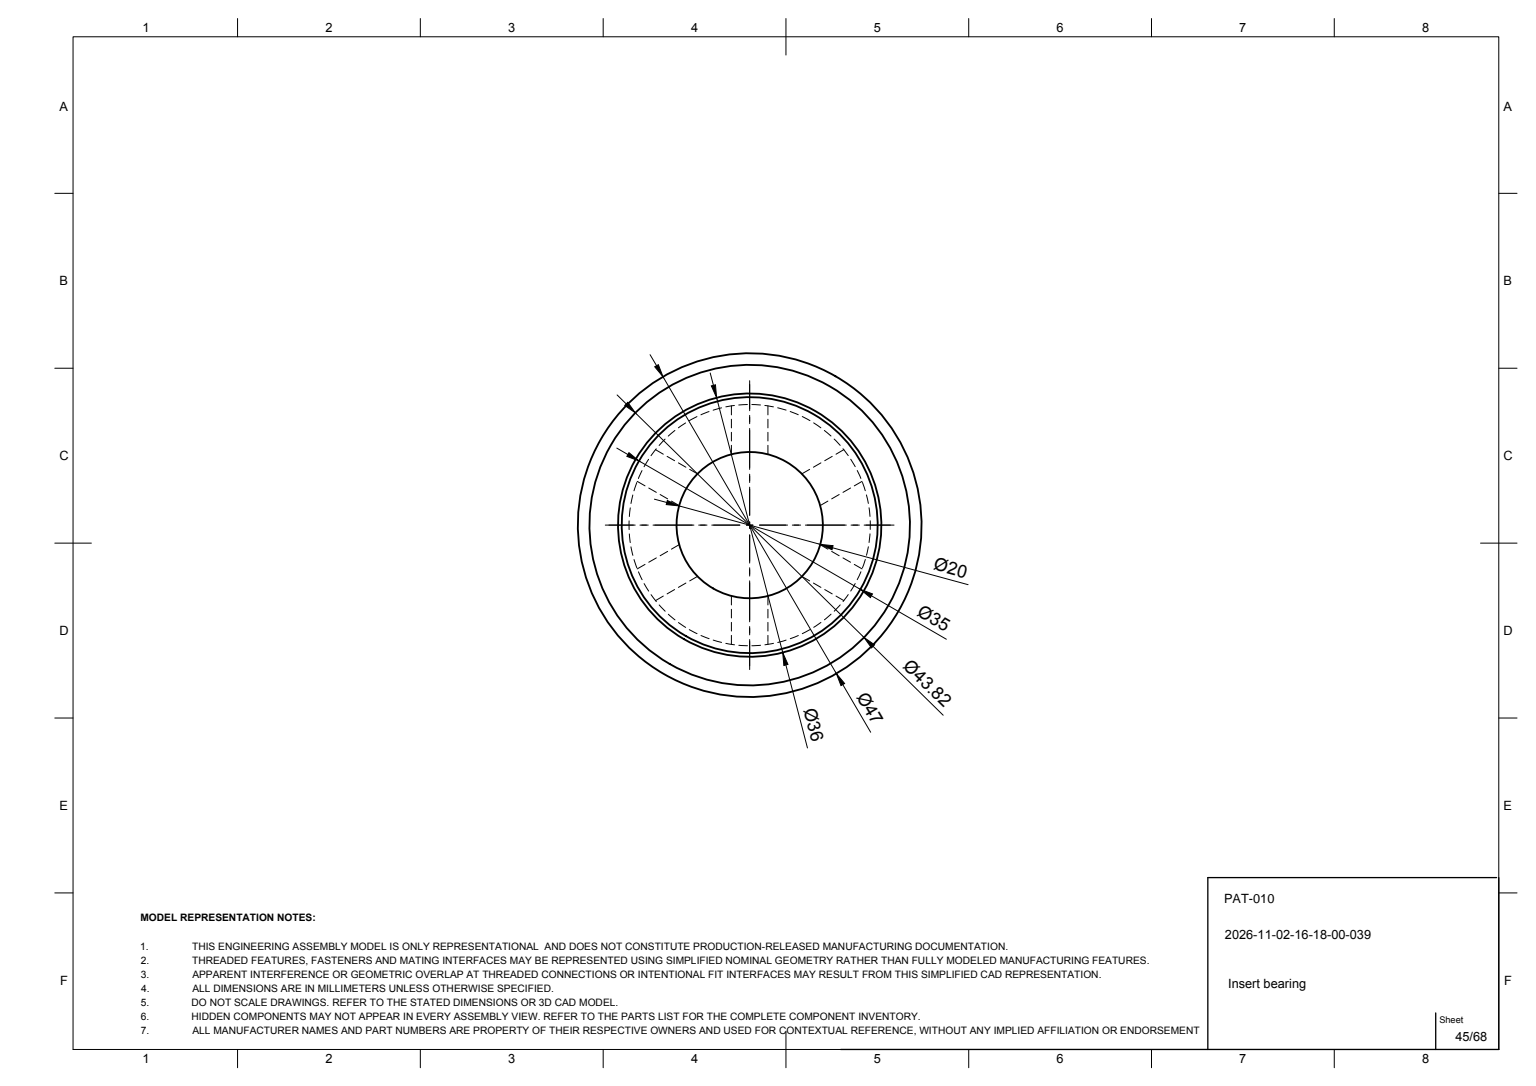
ISO-10303-21;
HEADER;
/* Generated by software containing ST-Developer
 * from STEP Tools, Inc. (www.steptools.com) 
 */

FILE_DESCRIPTION(
/* description */ ('Belt conveyor head drive unit'),
/* implementation_level */ '2;1');

FILE_NAME(
/* name */ 'Insert bearing.step',
/* time_stamp */ '2026-10-28T03:26:19-07:00',
/* author */ (''),
/* organization */ (''),
/* preprocessor_version */ 'ST-DEVELOPER v20.2',
/* originating_system */ 'Autodesk Translation Framework v15.17.0.0',
/* authorisation */ '');

FILE_SCHEMA (('AUTOMOTIVE_DESIGN { 1 0 10303 214 3 1 1 }'));
ENDSEC;

DATA;
#10=MECHANICAL_DESIGN_GEOMETRIC_PRESENTATION_REPRESENTATION('',(#902,#903),#27069);
#553=B_SPLINE_CURVE_WITH_KNOTS('',3,(#23805,#23806,#23807,#23808,#23809,
#23810,#23811,#23812,#23813,#23814),.UNSPECIFIED.,.F.,.F.,(4,2,2,2,4),(1.13193471301885,
1.22626174930539,1.32058878559194,1.41491753480854,1.50924628402513),
 .UNSPECIFIED.);
#554=B_SPLINE_CURVE_WITH_KNOTS('',3,(#23816,#23817,#23818,#23819,#23820,
#23821,#23822,#23823,#23824,#23825,#23826,#23827,#23828,#23829,#23830,#23831,
#23832,#23833),.UNSPECIFIED.,.F.,.F.,(4,2,2,2,2,2,2,2,4),(0.377311571006283,
0.471638607292829,0.565965643579376,0.66029439279597,0.754623142012565,
0.84895189122916,0.943280640445754,1.0376076767323,1.13193471301885),
 .UNSPECIFIED.);
#555=B_SPLINE_CURVE_WITH_KNOTS('',3,(#23834,#23835,#23836,#23837,#23838,
#23839,#23840,#23841,#23842,#23843),.UNSPECIFIED.,.F.,.F.,(4,2,2,2,4),(1.50924628402513,
1.60357503324173,1.69790378245832,1.79223081874487,1.88655785503141),
 .UNSPECIFIED.);
#556=B_SPLINE_CURVE_WITH_KNOTS('',3,(#23846,#23847,#23848,#23849,#23850,
#23851,#23852,#23853,#23854,#23855,#23856,#23857,#23858,#23859,#23860,#23861,
#23862,#23863,#23864,#23865,#23866,#23867,#23868,#23869,#23870,#23871,#23872,
#23873,#23874,#23875,#23876,#23877,#23878,#23879),.UNSPECIFIED.,.T.,.F.,
(4,2,2,2,2,2,2,2,2,2,2,2,2,2,2,2,4),(0.,0.0946120580087934,0.189224116017587,
0.283822945575014,0.378421775132442,0.47302060468987,0.567619434247297,
0.662231492256091,0.756843550264884,0.851455608273677,0.94606766628247,
1.0406664958399,1.13526532539733,1.22986415495475,1.32446298451218,1.41907504252097,
1.51368710052977),.UNSPECIFIED.);
#557=B_SPLINE_CURVE_WITH_KNOTS('',3,(#23882,#23883,#23884,#23885,#23886,
#23887,#23888,#23889,#23890,#23891,#23892,#23893,#23894,#23895,#23896,#23897,
#23898,#23899,#23900,#23901,#23902,#23903,#23904,#23905,#23906,#23907,#23908,
#23909,#23910,#23911,#23912,#23913,#23914,#23915),.UNSPECIFIED.,.T.,.F.,
(4,2,2,2,2,2,2,2,2,2,2,2,2,2,2,2,4),(0.,0.0946120580087934,0.189224116017587,
0.283822945575014,0.378421775132442,0.47302060468987,0.567619434247297,
0.66223149225609,0.756843550264884,0.851455608273677,0.94606766628247,1.0406664958399,
1.13526532539733,1.22986415495475,1.32446298451218,1.41907504252097,1.51368710052977),
 .UNSPECIFIED.);
#558=B_SPLINE_CURVE_WITH_KNOTS('',3,(#23919,#23920,#23921,#23922,#23923,
#23924,#23925,#23926,#23927,#23928),.UNSPECIFIED.,.F.,.F.,(4,2,2,2,4),(1.13193471301885,
1.22626174930539,1.32058878559194,1.41491753480854,1.50924628402513),
 .UNSPECIFIED.);
#559=B_SPLINE_CURVE_WITH_KNOTS('',3,(#23930,#23931,#23932,#23933,#23934,
#23935,#23936,#23937,#23938,#23939,#23940,#23941,#23942,#23943,#23944,#23945,
#23946,#23947),.UNSPECIFIED.,.F.,.F.,(4,2,2,2,2,2,2,2,4),(0.377311571006283,
0.47163860729283,0.565965643579376,0.660294392795971,0.754623142012565,
0.84895189122916,0.943280640445755,1.0376076767323,1.13193471301885),
 .UNSPECIFIED.);
#560=B_SPLINE_CURVE_WITH_KNOTS('',3,(#23948,#23949,#23950,#23951,#23952,
#23953,#23954,#23955,#23956,#23957),.UNSPECIFIED.,.F.,.F.,(4,2,2,2,4),(1.50924628402513,
1.60357503324173,1.69790378245832,1.79223081874487,1.88655785503141),
 .UNSPECIFIED.);
#561=B_SPLINE_CURVE_WITH_KNOTS('',3,(#23966,#23967,#23968,#23969,#23970,
#23971,#23972,#23973,#23974,#23975,#23976,#23977,#23978,#23979,#23980,#23981,
#23982,#23983),.UNSPECIFIED.,.F.,.F.,(4,2,2,2,2,2,2,2,4),(0.377311571006282,
0.471638607292829,0.565965643579376,0.660294392795971,0.754623142012565,
0.84895189122916,0.943280640445754,1.0376076767323,1.13193471301885),
 .UNSPECIFIED.);
#562=B_SPLINE_CURVE_WITH_KNOTS('',3,(#23985,#23986,#23987,#23988,#23989,
#23990,#23991,#23992,#23993,#23994),.UNSPECIFIED.,.F.,.F.,(4,2,2,2,4),(1.13193471301885,
1.22626174930539,1.32058878559194,1.41491753480854,1.50924628402513),
 .UNSPECIFIED.);
#563=B_SPLINE_CURVE_WITH_KNOTS('',3,(#23995,#23996,#23997,#23998,#23999,
#24000,#24001,#24002,#24003,#24004),.UNSPECIFIED.,.F.,.F.,(4,2,2,2,4),(1.50924628402513,
1.60357503324172,1.69790378245832,1.79223081874487,1.88655785503141),
 .UNSPECIFIED.);
#564=B_SPLINE_CURVE_WITH_KNOTS('',3,(#24007,#24008,#24009,#24010,#24011,
#24012,#24013,#24014,#24015,#24016,#24017,#24018,#24019,#24020,#24021,#24022,
#24023,#24024),.UNSPECIFIED.,.F.,.F.,(4,2,2,2,2,2,2,2,4),(0.377311571006283,
0.47163860729283,0.565965643579376,0.660294392795971,0.754623142012565,
0.84895189122916,0.943280640445754,1.0376076767323,1.13193471301885),
 .UNSPECIFIED.);
#565=B_SPLINE_CURVE_WITH_KNOTS('',3,(#24026,#24027,#24028,#24029,#24030,
#24031,#24032,#24033,#24034,#24035),.UNSPECIFIED.,.F.,.F.,(4,2,2,2,4),(1.13193471301885,
1.22626174930539,1.32058878559194,1.41491753480854,1.50924628402513),
 .UNSPECIFIED.);
#566=B_SPLINE_CURVE_WITH_KNOTS('',3,(#24036,#24037,#24038,#24039,#24040,
#24041,#24042,#24043,#24044,#24045),.UNSPECIFIED.,.F.,.F.,(4,2,2,2,4),(1.50924628402513,
1.60357503324173,1.69790378245832,1.79223081874487,1.88655785503141),
 .UNSPECIFIED.);
#567=B_SPLINE_CURVE_WITH_KNOTS('',3,(#24048,#24049,#24050,#24051,#24052,
#24053,#24054,#24055,#24056,#24057,#24058,#24059,#24060,#24061,#24062,#24063,
#24064,#24065),.UNSPECIFIED.,.F.,.F.,(4,2,2,2,2,2,2,2,4),(0.377311571006282,
0.471638607292829,0.565965643579376,0.66029439279597,0.754623142012565,
0.84895189122916,0.943280640445754,1.0376076767323,1.13193471301885),
 .UNSPECIFIED.);
#568=B_SPLINE_CURVE_WITH_KNOTS('',3,(#24067,#24068,#24069,#24070,#24071,
#24072,#24073,#24074,#24075,#24076),.UNSPECIFIED.,.F.,.F.,(4,2,2,2,4),(1.13193471301885,
1.22626174930539,1.32058878559194,1.41491753480854,1.50924628402513),
 .UNSPECIFIED.);
#569=B_SPLINE_CURVE_WITH_KNOTS('',3,(#24077,#24078,#24079,#24080,#24081,
#24082,#24083,#24084,#24085,#24086),.UNSPECIFIED.,.F.,.F.,(4,2,2,2,4),(1.50924628402513,
1.60357503324172,1.69790378245832,1.79223081874487,1.88655785503141),
 .UNSPECIFIED.);
#570=B_SPLINE_CURVE_WITH_KNOTS('',3,(#24089,#24090,#24091,#24092,#24093,
#24094,#24095,#24096,#24097,#24098,#24099,#24100,#24101,#24102,#24103,#24104,
#24105,#24106),.UNSPECIFIED.,.F.,.F.,(4,2,2,2,2,2,2,2,4),(0.377311571006283,
0.471638607292829,0.565965643579376,0.660294392795971,0.754623142012565,
0.84895189122916,0.943280640445755,1.0376076767323,1.13193471301885),
 .UNSPECIFIED.);
#571=B_SPLINE_CURVE_WITH_KNOTS('',3,(#24108,#24109,#24110,#24111,#24112,
#24113,#24114,#24115,#24116,#24117),.UNSPECIFIED.,.F.,.F.,(4,2,2,2,4),(1.13193471301885,
1.22626174930539,1.32058878559194,1.41491753480854,1.50924628402513),
 .UNSPECIFIED.);
#572=B_SPLINE_CURVE_WITH_KNOTS('',3,(#24118,#24119,#24120,#24121,#24122,
#24123,#24124,#24125,#24126,#24127),.UNSPECIFIED.,.F.,.F.,(4,2,2,2,4),(1.50924628402513,
1.60357503324172,1.69790378245832,1.79223081874487,1.88655785503141),
 .UNSPECIFIED.);
#573=B_SPLINE_CURVE_WITH_KNOTS('',3,(#24131,#24132,#24133,#24134,#24135,
#24136,#24137,#24138,#24139,#24140,#24141,#24142,#24143,#24144,#24145,#24146,
#24147,#24148,#24149,#24150,#24151,#24152,#24153,#24154,#24155,#24156,#24157,
#24158,#24159,#24160,#24161,#24162,#24163,#24164),.UNSPECIFIED.,.T.,.F.,
(4,2,2,2,2,2,2,2,2,2,2,2,2,2,2,2,4),(0.,0.0946120580087934,0.189224116017587,
0.283822945575014,0.378421775132442,0.47302060468987,0.567619434247297,
0.66223149225609,0.756843550264884,0.851455608273677,0.94606766628247,1.0406664958399,
1.13526532539733,1.22986415495475,1.32446298451218,1.41907504252097,1.51368710052977),
 .UNSPECIFIED.);
#574=B_SPLINE_CURVE_WITH_KNOTS('',3,(#24167,#24168,#24169,#24170,#24171,
#24172,#24173,#24174,#24175,#24176,#24177,#24178,#24179,#24180,#24181,#24182,
#24183,#24184,#24185,#24186,#24187,#24188,#24189,#24190,#24191,#24192,#24193,
#24194,#24195,#24196,#24197,#24198,#24199,#24200),.UNSPECIFIED.,.T.,.F.,
(4,2,2,2,2,2,2,2,2,2,2,2,2,2,2,2,4),(0.,0.0946120580087934,0.189224116017587,
0.283822945575014,0.378421775132442,0.47302060468987,0.567619434247297,
0.66223149225609,0.756843550264884,0.851455608273677,0.94606766628247,1.0406664958399,
1.13526532539733,1.22986415495475,1.32446298451218,1.41907504252097,1.51368710052977),
 .UNSPECIFIED.);
#575=B_SPLINE_CURVE_WITH_KNOTS('',3,(#24205,#24206,#24207,#24208,#24209,
#24210,#24211,#24212,#24213,#24214,#24215,#24216,#24217,#24218,#24219,#24220,
#24221,#24222,#24223,#24224,#24225,#24226,#24227,#24228,#24229,#24230,#24231,
#24232,#24233,#24234,#24235,#24236,#24237,#24238),.UNSPECIFIED.,.T.,.F.,
(4,2,2,2,2,2,2,2,2,2,2,2,2,2,2,2,4),(0.,0.0946120580087934,0.189224116017587,
0.283822945575014,0.378421775132442,0.47302060468987,0.567619434247297,
0.66223149225609,0.756843550264884,0.851455608273677,0.94606766628247,1.0406664958399,
1.13526532539733,1.22986415495475,1.32446298451218,1.41907504252097,1.51368710052977),
 .UNSPECIFIED.);
#576=B_SPLINE_CURVE_WITH_KNOTS('',3,(#24241,#24242,#24243,#24244,#24245,
#24246,#24247,#24248,#24249,#24250,#24251,#24252,#24253,#24254,#24255,#24256,
#24257,#24258,#24259,#24260,#24261,#24262,#24263,#24264,#24265,#24266,#24267,
#24268,#24269,#24270,#24271,#24272,#24273,#24274),.UNSPECIFIED.,.T.,.F.,
(4,2,2,2,2,2,2,2,2,2,2,2,2,2,2,2,4),(0.,0.0946120580087934,0.189224116017587,
0.283822945575014,0.378421775132442,0.47302060468987,0.567619434247297,
0.66223149225609,0.756843550264884,0.851455608273677,0.94606766628247,1.0406664958399,
1.13526532539733,1.22986415495475,1.32446298451218,1.41907504252097,1.51368710052977),
 .UNSPECIFIED.);
#676=SPHERICAL_SURFACE('',#15555,2.35);
#749=SHAPE_REPRESENTATION_RELATIONSHIP('SRR','None',#27396,#818);
#818=ADVANCED_BREP_SHAPE_REPRESENTATION('',(#985,#986),#27038);
#902=STYLED_ITEM('',(#27797),#985);
#903=STYLED_ITEM('',(#27797),#986);
#985=MANIFOLD_SOLID_BREP('Body1',#13769);
#986=MANIFOLD_SOLID_BREP('Body2',#13770);
#1182=FACE_BOUND('',#3067,.T.);
#1183=FACE_BOUND('',#3069,.T.);
#1184=FACE_BOUND('',#3070,.T.);
#1185=FACE_BOUND('',#3072,.T.);
#1186=FACE_BOUND('',#3076,.T.);
#1187=FACE_BOUND('',#3077,.T.);
#1188=FACE_BOUND('',#3078,.T.);
#1189=FACE_BOUND('',#3079,.T.);
#1190=FACE_BOUND('',#3080,.T.);
#1191=FACE_BOUND('',#3081,.T.);
#1192=FACE_BOUND('',#3087,.T.);
#1193=FACE_BOUND('',#3089,.T.);
#1194=FACE_BOUND('',#3092,.T.);
#1195=FACE_BOUND('',#3094,.T.);
#1196=FACE_BOUND('',#3095,.T.);
#1197=FACE_BOUND('',#3096,.T.);
#1198=FACE_BOUND('',#3097,.T.);
#1199=FACE_BOUND('',#3098,.T.);
#1200=FACE_BOUND('',#3099,.T.);
#1512=PLANE('',#15553);
#1513=PLANE('',#15558);
#1514=PLANE('',#15568);
#1515=PLANE('',#15570);
#1516=PLANE('',#15574);
#2095=FACE_OUTER_BOUND('',#3065,.T.);
#2096=FACE_OUTER_BOUND('',#3066,.T.);
#2097=FACE_OUTER_BOUND('',#3068,.T.);
#2098=FACE_OUTER_BOUND('',#3071,.T.);
#2099=FACE_OUTER_BOUND('',#3073,.T.);
#2100=FACE_OUTER_BOUND('',#3074,.T.);
#2101=FACE_OUTER_BOUND('',#3075,.T.);
#2102=FACE_OUTER_BOUND('',#3082,.T.);
#2103=FACE_OUTER_BOUND('',#3083,.T.);
#2104=FACE_OUTER_BOUND('',#3084,.T.);
#2105=FACE_OUTER_BOUND('',#3085,.T.);
#2106=FACE_OUTER_BOUND('',#3086,.T.);
#2107=FACE_OUTER_BOUND('',#3088,.T.);
#2108=FACE_OUTER_BOUND('',#3090,.T.);
#2109=FACE_OUTER_BOUND('',#3091,.T.);
#2110=FACE_OUTER_BOUND('',#3093,.T.);
#3065=EDGE_LOOP('',(#10938,#10939,#10940,#10941));
#3066=EDGE_LOOP('',(#10942));
#3067=EDGE_LOOP('',(#10943));
#3068=EDGE_LOOP('',(#10944,#10945));
#3069=EDGE_LOOP('',(#10946));
#3070=EDGE_LOOP('',(#10947));
#3071=EDGE_LOOP('',(#10948));
#3072=EDGE_LOOP('',(#10949));
#3073=EDGE_LOOP('',(#10950,#10951,#10952,#10953,#10954,#10955));
#3074=EDGE_LOOP('',(#10956,#10957,#10958,#10959,#10960,#10961));
#3075=EDGE_LOOP('',(#10962,#10963,#10964,#10965));
#3076=EDGE_LOOP('',(#10966,#10967,#10968));
#3077=EDGE_LOOP('',(#10969,#10970,#10971));
#3078=EDGE_LOOP('',(#10972,#10973,#10974));
#3079=EDGE_LOOP('',(#10975,#10976,#10977));
#3080=EDGE_LOOP('',(#10978,#10979,#10980));
#3081=EDGE_LOOP('',(#10981,#10982,#10983));
#3082=EDGE_LOOP('',(#10984,#10985,#10986,#10987,#10988,#10989));
#3083=EDGE_LOOP('',(#10990,#10991,#10992,#10993,#10994,#10995));
#3084=EDGE_LOOP('',(#10996,#10997,#10998,#10999,#11000,#11001));
#3085=EDGE_LOOP('',(#11002,#11003,#11004,#11005,#11006,#11007));
#3086=EDGE_LOOP('',(#11008));
#3087=EDGE_LOOP('',(#11009));
#3088=EDGE_LOOP('',(#11010));
#3089=EDGE_LOOP('',(#11011));
#3090=EDGE_LOOP('',(#11012,#11013,#11014,#11015));
#3091=EDGE_LOOP('',(#11016));
#3092=EDGE_LOOP('',(#11017));
#3093=EDGE_LOOP('',(#11018,#11019,#11020,#11021));
#3094=EDGE_LOOP('',(#11022));
#3095=EDGE_LOOP('',(#11023));
#3096=EDGE_LOOP('',(#11024));
#3097=EDGE_LOOP('',(#11025));
#3098=EDGE_LOOP('',(#11026));
#3099=EDGE_LOOP('',(#11027));
#3986=LINE('',#23790,#4778);
#3987=LINE('',#23845,#4779);
#3988=LINE('',#23917,#4780);
#3989=LINE('',#23962,#4781);
#3990=LINE('',#24130,#4782);
#3991=LINE('',#24201,#4783);
#3992=LINE('',#24204,#4784);
#3993=LINE('',#24275,#4785);
#3994=LINE('',#24285,#4786);
#3995=LINE('',#24290,#4787);
#4778=VECTOR('',#18902,1.8);
#4779=VECTOR('',#18919,0.25);
#4780=VECTOR('',#18922,0.25);
#4781=VECTOR('',#18927,1.65);
#4782=VECTOR('',#18932,0.25);
#4783=VECTOR('',#18935,0.25);
#4784=VECTOR('',#18938,0.25);
#4785=VECTOR('',#18941,0.25);
#4786=VECTOR('',#18954,1.75);
#4787=VECTOR('',#18961,1.);
#5552=CIRCLE('',#15551,1.8);
#5553=CIRCLE('',#15552,1.8);
#5554=CIRCLE('',#15554,2.19089023002066);
#5555=CIRCLE('',#15556,2.35);
#5556=CIRCLE('',#15557,2.19089023002066);
#5557=CIRCLE('',#15562,1.65);
#5558=CIRCLE('',#15563,1.65);
#5559=CIRCLE('',#15569,1.);
#5560=CIRCLE('',#15571,1.75);
#5561=CIRCLE('',#15573,1.75);
#5562=CIRCLE('',#15575,1.);
#6629=VERTEX_POINT('',#23787);
#6630=VERTEX_POINT('',#23789);
#6631=VERTEX_POINT('',#23793);
#6632=VERTEX_POINT('',#23796);
#6633=VERTEX_POINT('',#23797);
#6634=VERTEX_POINT('',#23799);
#6635=VERTEX_POINT('',#23803);
#6636=VERTEX_POINT('',#23804);
#6637=VERTEX_POINT('',#23815);
#6638=VERTEX_POINT('',#23844);
#6639=VERTEX_POINT('',#23881);
#6640=VERTEX_POINT('',#23916);
#6641=VERTEX_POINT('',#23918);
#6642=VERTEX_POINT('',#23929);
#6643=VERTEX_POINT('',#23959);
#6644=VERTEX_POINT('',#23961);
#6645=VERTEX_POINT('',#23964);
#6646=VERTEX_POINT('',#23965);
#6647=VERTEX_POINT('',#23984);
#6648=VERTEX_POINT('',#24005);
#6649=VERTEX_POINT('',#24006);
#6650=VERTEX_POINT('',#24025);
#6651=VERTEX_POINT('',#24046);
#6652=VERTEX_POINT('',#24047);
#6653=VERTEX_POINT('',#24066);
#6654=VERTEX_POINT('',#24087);
#6655=VERTEX_POINT('',#24088);
#6656=VERTEX_POINT('',#24107);
#6657=VERTEX_POINT('',#24129);
#6658=VERTEX_POINT('',#24166);
#6659=VERTEX_POINT('',#24203);
#6660=VERTEX_POINT('',#24240);
#6661=VERTEX_POINT('',#24277);
#6662=VERTEX_POINT('',#24280);
#6663=VERTEX_POINT('',#24283);
#6664=VERTEX_POINT('',#24287);
#8161=EDGE_CURVE('',#6629,#6629,#5552,.T.);
#8162=EDGE_CURVE('',#6629,#6630,#3986,.T.);
#8163=EDGE_CURVE('',#6630,#6630,#5553,.T.);
#8164=EDGE_CURVE('',#6631,#6631,#5554,.T.);
#8165=EDGE_CURVE('',#6632,#6633,#5555,.T.);
#8166=EDGE_CURVE('',#6634,#6634,#5556,.T.);
#8167=EDGE_CURVE('',#6635,#6636,#553,.T.);
#8168=EDGE_CURVE('',#6637,#6635,#554,.T.);
#8169=EDGE_CURVE('',#6636,#6637,#555,.T.);
#8170=EDGE_CURVE('',#6636,#6638,#3987,.T.);
#8171=EDGE_CURVE('',#6638,#6638,#556,.T.);
#8172=EDGE_CURVE('',#6639,#6639,#557,.T.);
#8173=EDGE_CURVE('',#6639,#6640,#3988,.T.);
#8174=EDGE_CURVE('',#6641,#6640,#558,.T.);
#8175=EDGE_CURVE('',#6642,#6641,#559,.T.);
#8176=EDGE_CURVE('',#6640,#6642,#560,.T.);
#8177=EDGE_CURVE('',#6643,#6643,#5557,.T.);
#8178=EDGE_CURVE('',#6643,#6644,#3989,.T.);
#8179=EDGE_CURVE('',#6644,#6644,#5558,.T.);
#8180=EDGE_CURVE('',#6645,#6646,#561,.T.);
#8181=EDGE_CURVE('',#6646,#6647,#562,.T.);
#8182=EDGE_CURVE('',#6647,#6645,#563,.T.);
#8183=EDGE_CURVE('',#6648,#6649,#564,.T.);
#8184=EDGE_CURVE('',#6649,#6650,#565,.T.);
#8185=EDGE_CURVE('',#6650,#6648,#566,.T.);
#8186=EDGE_CURVE('',#6651,#6652,#567,.T.);
#8187=EDGE_CURVE('',#6652,#6653,#568,.T.);
#8188=EDGE_CURVE('',#6653,#6651,#569,.T.);
#8189=EDGE_CURVE('',#6654,#6655,#570,.T.);
#8190=EDGE_CURVE('',#6655,#6656,#571,.T.);
#8191=EDGE_CURVE('',#6656,#6654,#572,.T.);
#8192=EDGE_CURVE('',#6647,#6657,#3990,.T.);
#8193=EDGE_CURVE('',#6657,#6657,#573,.T.);
#8194=EDGE_CURVE('',#6658,#6658,#574,.T.);
#8195=EDGE_CURVE('',#6658,#6650,#3991,.T.);
#8196=EDGE_CURVE('',#6653,#6659,#3992,.T.);
#8197=EDGE_CURVE('',#6659,#6659,#575,.T.);
#8198=EDGE_CURVE('',#6660,#6660,#576,.T.);
#8199=EDGE_CURVE('',#6660,#6656,#3993,.T.);
#8200=EDGE_CURVE('',#6661,#6661,#5559,.T.);
#8201=EDGE_CURVE('',#6662,#6662,#5560,.T.);
#8202=EDGE_CURVE('',#6663,#6663,#5561,.T.);
#8203=EDGE_CURVE('',#6663,#6662,#3994,.T.);
#8204=EDGE_CURVE('',#6664,#6664,#5562,.T.);
#8205=EDGE_CURVE('',#6664,#6661,#3995,.T.);
#10938=ORIENTED_EDGE('',*,*,#8161,.T.);
#10939=ORIENTED_EDGE('',*,*,#8162,.T.);
#10940=ORIENTED_EDGE('',*,*,#8163,.F.);
#10941=ORIENTED_EDGE('',*,*,#8162,.F.);
#10942=ORIENTED_EDGE('',*,*,#8164,.F.);
#10943=ORIENTED_EDGE('',*,*,#8163,.T.);
#10944=ORIENTED_EDGE('',*,*,#8165,.T.);
#10945=ORIENTED_EDGE('',*,*,#8165,.F.);
#10946=ORIENTED_EDGE('',*,*,#8164,.T.);
#10947=ORIENTED_EDGE('',*,*,#8166,.F.);
#10948=ORIENTED_EDGE('',*,*,#8166,.T.);
#10949=ORIENTED_EDGE('',*,*,#8161,.F.);
#10950=ORIENTED_EDGE('',*,*,#8167,.F.);
#10951=ORIENTED_EDGE('',*,*,#8168,.F.);
#10952=ORIENTED_EDGE('',*,*,#8169,.F.);
#10953=ORIENTED_EDGE('',*,*,#8170,.T.);
#10954=ORIENTED_EDGE('',*,*,#8171,.F.);
#10955=ORIENTED_EDGE('',*,*,#8170,.F.);
#10956=ORIENTED_EDGE('',*,*,#8172,.F.);
#10957=ORIENTED_EDGE('',*,*,#8173,.T.);
#10958=ORIENTED_EDGE('',*,*,#8174,.F.);
#10959=ORIENTED_EDGE('',*,*,#8175,.F.);
#10960=ORIENTED_EDGE('',*,*,#8176,.F.);
#10961=ORIENTED_EDGE('',*,*,#8173,.F.);
#10962=ORIENTED_EDGE('',*,*,#8177,.F.);
#10963=ORIENTED_EDGE('',*,*,#8178,.T.);
#10964=ORIENTED_EDGE('',*,*,#8179,.T.);
#10965=ORIENTED_EDGE('',*,*,#8178,.F.);
#10966=ORIENTED_EDGE('',*,*,#8168,.T.);
#10967=ORIENTED_EDGE('',*,*,#8167,.T.);
#10968=ORIENTED_EDGE('',*,*,#8169,.T.);
#10969=ORIENTED_EDGE('',*,*,#8175,.T.);
#10970=ORIENTED_EDGE('',*,*,#8174,.T.);
#10971=ORIENTED_EDGE('',*,*,#8176,.T.);
#10972=ORIENTED_EDGE('',*,*,#8180,.T.);
#10973=ORIENTED_EDGE('',*,*,#8181,.T.);
#10974=ORIENTED_EDGE('',*,*,#8182,.T.);
#10975=ORIENTED_EDGE('',*,*,#8183,.T.);
#10976=ORIENTED_EDGE('',*,*,#8184,.T.);
#10977=ORIENTED_EDGE('',*,*,#8185,.T.);
#10978=ORIENTED_EDGE('',*,*,#8186,.T.);
#10979=ORIENTED_EDGE('',*,*,#8187,.T.);
#10980=ORIENTED_EDGE('',*,*,#8188,.T.);
#10981=ORIENTED_EDGE('',*,*,#8189,.T.);
#10982=ORIENTED_EDGE('',*,*,#8190,.T.);
#10983=ORIENTED_EDGE('',*,*,#8191,.T.);
#10984=ORIENTED_EDGE('',*,*,#8181,.F.);
#10985=ORIENTED_EDGE('',*,*,#8180,.F.);
#10986=ORIENTED_EDGE('',*,*,#8182,.F.);
#10987=ORIENTED_EDGE('',*,*,#8192,.T.);
#10988=ORIENTED_EDGE('',*,*,#8193,.F.);
#10989=ORIENTED_EDGE('',*,*,#8192,.F.);
#10990=ORIENTED_EDGE('',*,*,#8194,.F.);
#10991=ORIENTED_EDGE('',*,*,#8195,.T.);
#10992=ORIENTED_EDGE('',*,*,#8184,.F.);
#10993=ORIENTED_EDGE('',*,*,#8183,.F.);
#10994=ORIENTED_EDGE('',*,*,#8185,.F.);
#10995=ORIENTED_EDGE('',*,*,#8195,.F.);
#10996=ORIENTED_EDGE('',*,*,#8187,.F.);
#10997=ORIENTED_EDGE('',*,*,#8186,.F.);
#10998=ORIENTED_EDGE('',*,*,#8188,.F.);
#10999=ORIENTED_EDGE('',*,*,#8196,.T.);
#11000=ORIENTED_EDGE('',*,*,#8197,.F.);
#11001=ORIENTED_EDGE('',*,*,#8196,.F.);
#11002=ORIENTED_EDGE('',*,*,#8198,.F.);
#11003=ORIENTED_EDGE('',*,*,#8199,.T.);
#11004=ORIENTED_EDGE('',*,*,#8190,.F.);
#11005=ORIENTED_EDGE('',*,*,#8189,.F.);
#11006=ORIENTED_EDGE('',*,*,#8191,.F.);
#11007=ORIENTED_EDGE('',*,*,#8199,.F.);
#11008=ORIENTED_EDGE('',*,*,#8179,.F.);
#11009=ORIENTED_EDGE('',*,*,#8200,.T.);
#11010=ORIENTED_EDGE('',*,*,#8201,.F.);
#11011=ORIENTED_EDGE('',*,*,#8177,.T.);
#11012=ORIENTED_EDGE('',*,*,#8202,.F.);
#11013=ORIENTED_EDGE('',*,*,#8203,.T.);
#11014=ORIENTED_EDGE('',*,*,#8201,.T.);
#11015=ORIENTED_EDGE('',*,*,#8203,.F.);
#11016=ORIENTED_EDGE('',*,*,#8202,.T.);
#11017=ORIENTED_EDGE('',*,*,#8204,.F.);
#11018=ORIENTED_EDGE('',*,*,#8204,.T.);
#11019=ORIENTED_EDGE('',*,*,#8205,.T.);
#11020=ORIENTED_EDGE('',*,*,#8200,.F.);
#11021=ORIENTED_EDGE('',*,*,#8205,.F.);
#11022=ORIENTED_EDGE('',*,*,#8172,.T.);
#11023=ORIENTED_EDGE('',*,*,#8171,.T.);
#11024=ORIENTED_EDGE('',*,*,#8194,.T.);
#11025=ORIENTED_EDGE('',*,*,#8193,.T.);
#11026=ORIENTED_EDGE('',*,*,#8198,.T.);
#11027=ORIENTED_EDGE('',*,*,#8197,.T.);
#12708=CYLINDRICAL_SURFACE('',#15550,1.8);
#12709=CYLINDRICAL_SURFACE('',#15559,0.25);
#12710=CYLINDRICAL_SURFACE('',#15560,0.25);
#12711=CYLINDRICAL_SURFACE('',#15561,1.65);
#12712=CYLINDRICAL_SURFACE('',#15564,0.25);
#12713=CYLINDRICAL_SURFACE('',#15565,0.25);
#12714=CYLINDRICAL_SURFACE('',#15566,0.25);
#12715=CYLINDRICAL_SURFACE('',#15567,0.25);
#12716=CYLINDRICAL_SURFACE('',#15572,1.75);
#12717=CYLINDRICAL_SURFACE('',#15576,1.);
#13374=ADVANCED_FACE('',(#2095),#12708,.F.);
#13375=ADVANCED_FACE('',(#2096,#1182),#1512,.T.);
#13376=ADVANCED_FACE('',(#2097,#1183,#1184),#676,.T.);
#13377=ADVANCED_FACE('',(#2098,#1185),#1513,.T.);
#13378=ADVANCED_FACE('',(#2099),#12709,.F.);
#13379=ADVANCED_FACE('',(#2100),#12710,.F.);
#13380=ADVANCED_FACE('',(#2101,#1186,#1187,#1188,#1189,#1190,#1191),#12711,
 .T.);
#13381=ADVANCED_FACE('',(#2102),#12712,.F.);
#13382=ADVANCED_FACE('',(#2103),#12713,.F.);
#13383=ADVANCED_FACE('',(#2104),#12714,.F.);
#13384=ADVANCED_FACE('',(#2105),#12715,.F.);
#13385=ADVANCED_FACE('',(#2106,#1192),#1514,.T.);
#13386=ADVANCED_FACE('',(#2107,#1193),#1515,.T.);
#13387=ADVANCED_FACE('',(#2108),#12716,.T.);
#13388=ADVANCED_FACE('',(#2109,#1194),#1516,.T.);
#13389=ADVANCED_FACE('',(#2110,#1195,#1196,#1197,#1198,#1199,#1200),#12717,
 .F.);
#13769=CLOSED_SHELL('',(#13374,#13375,#13376,#13377));
#13770=CLOSED_SHELL('',(#13378,#13379,#13380,#13381,#13382,#13383,#13384,
#13385,#13386,#13387,#13388,#13389));
#15549=AXIS2_PLACEMENT_3D('',#23785,#18896,#18897);
#15550=AXIS2_PLACEMENT_3D('',#23786,#18898,#18899);
#15551=AXIS2_PLACEMENT_3D('',#23788,#18900,#18901);
#15552=AXIS2_PLACEMENT_3D('',#23791,#18903,#18904);
#15553=AXIS2_PLACEMENT_3D('',#23792,#18905,#18906);
#15554=AXIS2_PLACEMENT_3D('',#23794,#18907,#18908);
#15555=AXIS2_PLACEMENT_3D('',#23795,#18909,#18910);
#15556=AXIS2_PLACEMENT_3D('',#23798,#18911,#18912);
#15557=AXIS2_PLACEMENT_3D('',#23800,#18913,#18914);
#15558=AXIS2_PLACEMENT_3D('',#23801,#18915,#18916);
#15559=AXIS2_PLACEMENT_3D('',#23802,#18917,#18918);
#15560=AXIS2_PLACEMENT_3D('',#23880,#18920,#18921);
#15561=AXIS2_PLACEMENT_3D('',#23958,#18923,#18924);
#15562=AXIS2_PLACEMENT_3D('',#23960,#18925,#18926);
#15563=AXIS2_PLACEMENT_3D('',#23963,#18928,#18929);
#15564=AXIS2_PLACEMENT_3D('',#24128,#18930,#18931);
#15565=AXIS2_PLACEMENT_3D('',#24165,#18933,#18934);
#15566=AXIS2_PLACEMENT_3D('',#24202,#18936,#18937);
#15567=AXIS2_PLACEMENT_3D('',#24239,#18939,#18940);
#15568=AXIS2_PLACEMENT_3D('',#24276,#18942,#18943);
#15569=AXIS2_PLACEMENT_3D('',#24278,#18944,#18945);
#15570=AXIS2_PLACEMENT_3D('',#24279,#18946,#18947);
#15571=AXIS2_PLACEMENT_3D('',#24281,#18948,#18949);
#15572=AXIS2_PLACEMENT_3D('',#24282,#18950,#18951);
#15573=AXIS2_PLACEMENT_3D('',#24284,#18952,#18953);
#15574=AXIS2_PLACEMENT_3D('',#24286,#18955,#18956);
#15575=AXIS2_PLACEMENT_3D('',#24288,#18957,#18958);
#15576=AXIS2_PLACEMENT_3D('',#24289,#18959,#18960);
#18896=DIRECTION('axis',(0.,0.,1.));
#18897=DIRECTION('refdir',(1.,0.,0.));
#18898=DIRECTION('center_axis',(0.,-1.,0.));
#18899=DIRECTION('ref_axis',(1.,0.,0.));
#18900=DIRECTION('center_axis',(0.,-1.,0.));
#18901=DIRECTION('ref_axis',(1.,0.,0.));
#18902=DIRECTION('',(0.,1.,0.));
#18903=DIRECTION('center_axis',(0.,-1.,0.));
#18904=DIRECTION('ref_axis',(1.,0.,0.));
#18905=DIRECTION('center_axis',(0.,1.,0.));
#18906=DIRECTION('ref_axis',(0.,0.,1.));
#18907=DIRECTION('center_axis',(0.,-1.,0.));
#18908=DIRECTION('ref_axis',(1.,0.,0.));
#18909=DIRECTION('center_axis',(6.12323399573677E-17,0.,1.));
#18910=DIRECTION('ref_axis',(1.,0.,0.));
#18911=DIRECTION('center_axis',(1.22464679914735E-16,-1.,0.));
#18912=DIRECTION('ref_axis',(-1.,-1.22464679914735E-16,0.));
#18913=DIRECTION('center_axis',(0.,-1.,0.));
#18914=DIRECTION('ref_axis',(1.,0.,0.));
#18915=DIRECTION('center_axis',(0.,-1.,0.));
#18916=DIRECTION('ref_axis',(0.,0.,-1.));
#18917=DIRECTION('center_axis',(-0.866025403784438,0.,-0.5));
#18918=DIRECTION('ref_axis',(-0.5,0.,0.866025403784438));
#18919=DIRECTION('',(-0.866025403784438,0.,-0.5));
#18920=DIRECTION('center_axis',(-0.866025403784438,0.,-0.5));
#18921=DIRECTION('ref_axis',(-0.5,0.,0.866025403784438));
#18922=DIRECTION('',(-0.866025403784438,0.,-0.5));
#18923=DIRECTION('center_axis',(0.,-1.,0.));
#18924=DIRECTION('ref_axis',(1.,0.,0.));
#18925=DIRECTION('center_axis',(0.,-1.,0.));
#18926=DIRECTION('ref_axis',(1.,0.,0.));
#18927=DIRECTION('',(0.,1.,0.));
#18928=DIRECTION('center_axis',(0.,-1.,0.));
#18929=DIRECTION('ref_axis',(1.,0.,0.));
#18930=DIRECTION('center_axis',(0.866025403784439,0.,-0.5));
#18931=DIRECTION('ref_axis',(-0.5,0.,-0.866025403784439));
#18932=DIRECTION('',(0.866025403784439,0.,-0.5));
#18933=DIRECTION('center_axis',(0.866025403784439,0.,-0.5));
#18934=DIRECTION('ref_axis',(-0.5,0.,-0.866025403784439));
#18935=DIRECTION('',(0.866025403784439,0.,-0.5));
#18936=DIRECTION('center_axis',(0.,0.,1.));
#18937=DIRECTION('ref_axis',(1.,0.,0.));
#18938=DIRECTION('',(0.,0.,1.));
#18939=DIRECTION('center_axis',(0.,0.,1.));
#18940=DIRECTION('ref_axis',(1.,0.,0.));
#18941=DIRECTION('',(0.,0.,1.));
#18942=DIRECTION('center_axis',(0.,1.,0.));
#18943=DIRECTION('ref_axis',(0.,0.,1.));
#18944=DIRECTION('center_axis',(0.,-1.,0.));
#18945=DIRECTION('ref_axis',(1.,0.,0.));
#18946=DIRECTION('center_axis',(0.,1.,0.));
#18947=DIRECTION('ref_axis',(0.,0.,1.));
#18948=DIRECTION('center_axis',(0.,-1.,0.));
#18949=DIRECTION('ref_axis',(1.,0.,0.));
#18950=DIRECTION('center_axis',(0.,-1.,0.));
#18951=DIRECTION('ref_axis',(1.,0.,0.));
#18952=DIRECTION('center_axis',(0.,-1.,0.));
#18953=DIRECTION('ref_axis',(1.,0.,0.));
#18954=DIRECTION('',(0.,1.,0.));
#18955=DIRECTION('center_axis',(0.,-1.,0.));
#18956=DIRECTION('ref_axis',(0.,0.,-1.));
#18957=DIRECTION('center_axis',(0.,-1.,0.));
#18958=DIRECTION('ref_axis',(1.,0.,0.));
#18959=DIRECTION('center_axis',(0.,-1.,0.));
#18960=DIRECTION('ref_axis',(1.,0.,0.));
#18961=DIRECTION('',(0.,1.,0.));
#23785=CARTESIAN_POINT('',(0.,0.,0.));
#23786=CARTESIAN_POINT('Origin',(0.,0.,0.));
#23787=CARTESIAN_POINT('',(-1.8,-0.85,-2.20436423846524E-16));
#23788=CARTESIAN_POINT('Origin',(0.,-0.85,0.));
#23789=CARTESIAN_POINT('',(-1.8,0.85,-2.20436423846524E-16));
#23790=CARTESIAN_POINT('',(-1.8,0.,-2.20436423846524E-16));
#23791=CARTESIAN_POINT('Origin',(0.,0.85,0.));
#23792=CARTESIAN_POINT('Origin',(2.19089023002066,0.85,0.));
#23793=CARTESIAN_POINT('',(2.19089023002066,0.85,0.));
#23794=CARTESIAN_POINT('Origin',(0.,0.85,0.));
#23795=CARTESIAN_POINT('Origin',(3.99680288865056E-15,0.,0.));
#23796=CARTESIAN_POINT('',(3.85290688975075E-15,-1.76221774462768E-32,2.35));
#23797=CARTESIAN_POINT('',(3.85290688975075E-15,-1.76221774462768E-32,-2.35));
#23798=CARTESIAN_POINT('Origin',(3.99680288865056E-15,0.,0.));
#23799=CARTESIAN_POINT('',(2.19089023002066,-0.85,0.));
#23800=CARTESIAN_POINT('Origin',(0.,-0.85,0.));
#23801=CARTESIAN_POINT('Origin',(1.8,-0.85,0.));
#23802=CARTESIAN_POINT('Origin',(0.,1.55,0.));
#23803=CARTESIAN_POINT('',(1.42894191624432,1.8,0.825000000000001));
#23804=CARTESIAN_POINT('',(1.53744468918255,1.55,0.598968970568896));
#23805=CARTESIAN_POINT('Ctrl Pts',(1.42894191624432,1.8,0.825000000000001));
#23806=CARTESIAN_POINT('Ctrl Pts',(1.44466308895875,1.8,0.797770130104052));
#23807=CARTESIAN_POINT('Ctrl Pts',(1.46055812562105,1.79370633789704,0.768258557763732));
#23808=CARTESIAN_POINT('Ctrl Pts',(1.48824888379079,1.76817777258318,0.713138492740816));
#23809=CARTESIAN_POINT('Ctrl Pts',(1.50008999307766,1.74894552961493,0.687551581002689));
#23810=CARTESIAN_POINT('Ctrl Pts',(1.51812136280714,1.70460745840382,0.646764802471699));
#23811=CARTESIAN_POINT('Ctrl Pts',(1.52552758004446,1.67652816181843,0.628833667319578));
#23812=CARTESIAN_POINT('Ctrl Pts',(1.53516661651472,1.61494799959182,0.604921184808251));
#23813=CARTESIAN_POINT('Ctrl Pts',(1.53744468918255,1.58144291640553,0.598968970568896));
#23814=CARTESIAN_POINT('Ctrl Pts',(1.53744468918255,1.55,0.598968970568896));
#23815=CARTESIAN_POINT('',(1.42894191624432,1.3,0.825000000000001));
#23816=CARTESIAN_POINT('Ctrl Pts',(1.42894191624432,1.3,0.825000000000001));
#23817=CARTESIAN_POINT('Ctrl Pts',(1.4132207435299,1.3,0.852229869895949));
#23818=CARTESIAN_POINT('Ctrl Pts',(1.39561049050871,1.30629366210296,0.880751161609749));
#23819=CARTESIAN_POINT('Ctrl Pts',(1.36172049302549,1.33182222741682,0.932292094146256));
#23820=CARTESIAN_POINT('Ctrl Pts',(1.34548213209931,1.35105447038507,0.955340251466734));
#23821=CARTESIAN_POINT('Ctrl Pts',(1.31917543061769,1.39539254159618,0.99134926498299));
#23822=CARTESIAN_POINT('Ctrl Pts',(1.30734972067592,1.42347183818157,1.00672880483252));
#23823=CARTESIAN_POINT('Ctrl Pts',(1.29146042158868,1.48505200040818,1.02703269653942));
#23824=CARTESIAN_POINT('Ctrl Pts',(1.28744468918255,1.51855708359447,1.03198167246111));
#23825=CARTESIAN_POINT('Ctrl Pts',(1.28744468918255,1.58144291640553,1.03198167246111));
#23826=CARTESIAN_POINT('Ctrl Pts',(1.29146042158868,1.61494799959182,1.02703269653942));
#23827=CARTESIAN_POINT('Ctrl Pts',(1.30734972067592,1.67652816181843,1.00672880483252));
#23828=CARTESIAN_POINT('Ctrl Pts',(1.31917543061769,1.70460745840382,0.991349264982991));
#23829=CARTESIAN_POINT('Ctrl Pts',(1.34548213209931,1.74894552961493,0.955340251466735));
#23830=CARTESIAN_POINT('Ctrl Pts',(1.36172049302549,1.76817777258318,0.932292094146256));
#23831=CARTESIAN_POINT('Ctrl Pts',(1.39561049050871,1.79370633789704,0.880751161609749));
#23832=CARTESIAN_POINT('Ctrl Pts',(1.4132207435299,1.8,0.85222986989595));
#23833=CARTESIAN_POINT('Ctrl Pts',(1.42894191624432,1.8,0.825000000000001));
#23834=CARTESIAN_POINT('Ctrl Pts',(1.53744468918255,1.55,0.598968970568896));
#23835=CARTESIAN_POINT('Ctrl Pts',(1.53744468918255,1.51855708359447,0.598968970568896));
#23836=CARTESIAN_POINT('Ctrl Pts',(1.53516661651472,1.48505200040818,0.60492118480825));
#23837=CARTESIAN_POINT('Ctrl Pts',(1.52552758004446,1.42347183818157,0.628833667319578));
#23838=CARTESIAN_POINT('Ctrl Pts',(1.51812136280714,1.39539254159618,0.646764802471699));
#23839=CARTESIAN_POINT('Ctrl Pts',(1.50008999307766,1.35105447038507,0.687551581002689));
#23840=CARTESIAN_POINT('Ctrl Pts',(1.48824888379079,1.33182222741682,0.713138492740816));
#23841=CARTESIAN_POINT('Ctrl Pts',(1.46055812562105,1.30629366210296,0.768258557763732));
#23842=CARTESIAN_POINT('Ctrl Pts',(1.44466308895875,1.3,0.797770130104052));
#23843=CARTESIAN_POINT('Ctrl Pts',(1.42894191624432,1.3,0.825000000000001));
#23844=CARTESIAN_POINT('',(0.963525491562421,1.55,0.267616567329818));
#23845=CARTESIAN_POINT('',(0.125,1.55,-0.21650635094611));
#23846=CARTESIAN_POINT('Ctrl Pts',(0.963525491562421,1.55,0.267616567329818));
#23847=CARTESIAN_POINT('Ctrl Pts',(0.963525491562421,1.5815373526696,0.267616567329818));
#23848=CARTESIAN_POINT('Ctrl Pts',(0.961833761492987,1.61508042700263,0.273949373987484));
#23849=CARTESIAN_POINT('Ctrl Pts',(0.954308486908894,1.67663267125761,0.299111603474268));
#23850=CARTESIAN_POINT('Ctrl Pts',(0.948394987258249,1.70465411363682,0.31788699900678));
#23851=CARTESIAN_POINT('Ctrl Pts',(0.933155485613026,1.74889618382539,0.360174810895352));
#23852=CARTESIAN_POINT('Ctrl Pts',(0.92278792026947,1.76811531482682,0.386546956384144));
#23853=CARTESIAN_POINT('Ctrl Pts',(0.897143218189782,1.79367084275751,0.442820664919227));
#23854=CARTESIAN_POINT('Ctrl Pts',(0.881791875377343,1.8,0.472691670144998));
#23855=CARTESIAN_POINT('Ctrl Pts',(0.850258932191534,1.8,0.527308329855003));
#23856=CARTESIAN_POINT('Ctrl Pts',(0.832065554235658,1.79367084275751,0.555538485325664));
#23857=CARTESIAN_POINT('Ctrl Pts',(0.796153444118959,1.76811531482682,0.605884303066698));
#23858=CARTESIAN_POINT('Ctrl Pts',(0.778498278845144,1.74889618382539,0.62804895077401));
#23859=CARTESIAN_POINT('Ctrl Pts',(0.749495710301794,1.70465411363682,0.662390652284073));
#23860=CARTESIAN_POINT('Ctrl Pts',(0.73619249062986,1.67663267125761,0.676899590973058));
#23861=CARTESIAN_POINT('Ctrl Pts',(0.718163997970498,1.61508042700263,0.695997784676728));
#23862=CARTESIAN_POINT('Ctrl Pts',(0.713525491562421,1.5815373526696,0.700629269222037));
#23863=CARTESIAN_POINT('Ctrl Pts',(0.713525491562421,1.5184626473304,0.700629269222037));
#23864=CARTESIAN_POINT('Ctrl Pts',(0.718163997970498,1.48491957299737,0.695997784676728));
#23865=CARTESIAN_POINT('Ctrl Pts',(0.73619249062986,1.42336732874239,0.676899590973058));
#23866=CARTESIAN_POINT('Ctrl Pts',(0.749495710301794,1.39534588636318,0.662390652284073));
#23867=CARTESIAN_POINT('Ctrl Pts',(0.778498278845144,1.35110381617461,0.62804895077401));
#23868=CARTESIAN_POINT('Ctrl Pts',(0.796153444118959,1.33188468517318,0.605884303066698));
#23869=CARTESIAN_POINT('Ctrl Pts',(0.832065554235658,1.30632915724249,0.555538485325664));
#23870=CARTESIAN_POINT('Ctrl Pts',(0.850258932191534,1.3,0.527308329855003));
#23871=CARTESIAN_POINT('Ctrl Pts',(0.881791875377343,1.3,0.472691670144998));
#23872=CARTESIAN_POINT('Ctrl Pts',(0.897143218189782,1.30632915724249,0.442820664919227));
#23873=CARTESIAN_POINT('Ctrl Pts',(0.92278792026947,1.33188468517318,0.386546956384144));
#23874=CARTESIAN_POINT('Ctrl Pts',(0.933155485613026,1.35110381617461,0.360174810895352));
#23875=CARTESIAN_POINT('Ctrl Pts',(0.948394987258249,1.39534588636318,0.31788699900678));
#23876=CARTESIAN_POINT('Ctrl Pts',(0.954308486908894,1.42336732874239,0.299111603474268));
#23877=CARTESIAN_POINT('Ctrl Pts',(0.961833761492987,1.48491957299738,0.273949373987484));
#23878=CARTESIAN_POINT('Ctrl Pts',(0.963525491562421,1.5184626473304,0.267616567329818));
#23879=CARTESIAN_POINT('Ctrl Pts',(0.963525491562421,1.55,0.267616567329818));
#23880=CARTESIAN_POINT('Origin',(0.,1.55,0.));
#23881=CARTESIAN_POINT('',(-0.713525491562421,1.55,-0.700629269222037));
#23882=CARTESIAN_POINT('Ctrl Pts',(-0.713525491562421,1.55,-0.700629269222037));
#23883=CARTESIAN_POINT('Ctrl Pts',(-0.713525491562421,1.5184626473304,-0.700629269222037));
#23884=CARTESIAN_POINT('Ctrl Pts',(-0.718163997970498,1.48491957299737,
-0.695997784676728));
#23885=CARTESIAN_POINT('Ctrl Pts',(-0.73619249062986,1.42336732874239,-0.676899590973058));
#23886=CARTESIAN_POINT('Ctrl Pts',(-0.749495710301794,1.39534588636318,
-0.662390652284073));
#23887=CARTESIAN_POINT('Ctrl Pts',(-0.778498278845144,1.35110381617461,
-0.62804895077401));
#23888=CARTESIAN_POINT('Ctrl Pts',(-0.796153444118959,1.33188468517318,
-0.605884303066698));
#23889=CARTESIAN_POINT('Ctrl Pts',(-0.832065554235658,1.30632915724249,
-0.555538485325664));
#23890=CARTESIAN_POINT('Ctrl Pts',(-0.850258932191534,1.3,-0.527308329855003));
#23891=CARTESIAN_POINT('Ctrl Pts',(-0.881791875377343,1.3,-0.472691670144998));
#23892=CARTESIAN_POINT('Ctrl Pts',(-0.897143218189782,1.30632915724249,
-0.442820664919227));
#23893=CARTESIAN_POINT('Ctrl Pts',(-0.92278792026947,1.33188468517318,-0.386546956384144));
#23894=CARTESIAN_POINT('Ctrl Pts',(-0.933155485613026,1.35110381617461,
-0.360174810895352));
#23895=CARTESIAN_POINT('Ctrl Pts',(-0.948394987258249,1.39534588636318,
-0.31788699900678));
#23896=CARTESIAN_POINT('Ctrl Pts',(-0.954308486908894,1.42336732874239,
-0.299111603474268));
#23897=CARTESIAN_POINT('Ctrl Pts',(-0.961833761492986,1.48491957299737,
-0.273949373987484));
#23898=CARTESIAN_POINT('Ctrl Pts',(-0.963525491562421,1.5184626473304,-0.267616567329818));
#23899=CARTESIAN_POINT('Ctrl Pts',(-0.963525491562421,1.5815373526696,-0.267616567329818));
#23900=CARTESIAN_POINT('Ctrl Pts',(-0.961833761492986,1.61508042700263,
-0.273949373987484));
#23901=CARTESIAN_POINT('Ctrl Pts',(-0.954308486908894,1.67663267125761,
-0.299111603474268));
#23902=CARTESIAN_POINT('Ctrl Pts',(-0.948394987258249,1.70465411363682,
-0.31788699900678));
#23903=CARTESIAN_POINT('Ctrl Pts',(-0.933155485613026,1.74889618382539,
-0.360174810895352));
#23904=CARTESIAN_POINT('Ctrl Pts',(-0.92278792026947,1.76811531482682,-0.386546956384144));
#23905=CARTESIAN_POINT('Ctrl Pts',(-0.897143218189782,1.79367084275751,
-0.442820664919227));
#23906=CARTESIAN_POINT('Ctrl Pts',(-0.881791875377343,1.8,-0.472691670144998));
#23907=CARTESIAN_POINT('Ctrl Pts',(-0.850258932191534,1.8,-0.527308329855003));
#23908=CARTESIAN_POINT('Ctrl Pts',(-0.832065554235658,1.79367084275751,
-0.555538485325664));
#23909=CARTESIAN_POINT('Ctrl Pts',(-0.796153444118959,1.76811531482682,
-0.605884303066698));
#23910=CARTESIAN_POINT('Ctrl Pts',(-0.778498278845144,1.74889618382539,
-0.62804895077401));
#23911=CARTESIAN_POINT('Ctrl Pts',(-0.749495710301794,1.70465411363682,
-0.662390652284073));
#23912=CARTESIAN_POINT('Ctrl Pts',(-0.73619249062986,1.67663267125761,-0.676899590973058));
#23913=CARTESIAN_POINT('Ctrl Pts',(-0.718163997970498,1.61508042700263,
-0.695997784676728));
#23914=CARTESIAN_POINT('Ctrl Pts',(-0.713525491562421,1.5815373526696,-0.700629269222037));
#23915=CARTESIAN_POINT('Ctrl Pts',(-0.713525491562421,1.55,-0.700629269222037));
#23916=CARTESIAN_POINT('',(-1.28744468918255,1.55,-1.03198167246111));
#23917=CARTESIAN_POINT('',(0.125,1.55,-0.21650635094611));
#23918=CARTESIAN_POINT('',(-1.42894191624432,1.3,-0.825000000000001));
#23919=CARTESIAN_POINT('Ctrl Pts',(-1.42894191624432,1.3,-0.825000000000001));
#23920=CARTESIAN_POINT('Ctrl Pts',(-1.4132207435299,1.3,-0.852229869895949));
#23921=CARTESIAN_POINT('Ctrl Pts',(-1.39561049050871,1.30629366210296,-0.880751161609749));
#23922=CARTESIAN_POINT('Ctrl Pts',(-1.36172049302549,1.33182222741682,-0.932292094146256));
#23923=CARTESIAN_POINT('Ctrl Pts',(-1.34548213209931,1.35105447038507,-0.955340251466735));
#23924=CARTESIAN_POINT('Ctrl Pts',(-1.31917543061769,1.39539254159618,-0.991349264982991));
#23925=CARTESIAN_POINT('Ctrl Pts',(-1.30734972067592,1.42347183818157,-1.00672880483252));
#23926=CARTESIAN_POINT('Ctrl Pts',(-1.29146042158868,1.48505200040818,-1.02703269653942));
#23927=CARTESIAN_POINT('Ctrl Pts',(-1.28744468918255,1.51855708359447,-1.03198167246111));
#23928=CARTESIAN_POINT('Ctrl Pts',(-1.28744468918255,1.55,-1.03198167246111));
#23929=CARTESIAN_POINT('',(-1.42894191624432,1.8,-0.825000000000001));
#23930=CARTESIAN_POINT('Ctrl Pts',(-1.42894191624432,1.8,-0.825000000000001));
#23931=CARTESIAN_POINT('Ctrl Pts',(-1.44466308895875,1.8,-0.797770130104052));
#23932=CARTESIAN_POINT('Ctrl Pts',(-1.46055812562105,1.79370633789704,-0.768258557763732));
#23933=CARTESIAN_POINT('Ctrl Pts',(-1.48824888379079,1.76817777258318,-0.713138492740816));
#23934=CARTESIAN_POINT('Ctrl Pts',(-1.50008999307766,1.74894552961493,-0.687551581002689));
#23935=CARTESIAN_POINT('Ctrl Pts',(-1.51812136280714,1.70460745840382,-0.646764802471699));
#23936=CARTESIAN_POINT('Ctrl Pts',(-1.52552758004446,1.67652816181843,-0.628833667319578));
#23937=CARTESIAN_POINT('Ctrl Pts',(-1.53516661651472,1.61494799959182,-0.60492118480825));
#23938=CARTESIAN_POINT('Ctrl Pts',(-1.53744468918255,1.58144291640553,-0.598968970568896));
#23939=CARTESIAN_POINT('Ctrl Pts',(-1.53744468918255,1.51855708359447,-0.598968970568896));
#23940=CARTESIAN_POINT('Ctrl Pts',(-1.53516661651472,1.48505200040818,-0.60492118480825));
#23941=CARTESIAN_POINT('Ctrl Pts',(-1.52552758004446,1.42347183818157,-0.628833667319578));
#23942=CARTESIAN_POINT('Ctrl Pts',(-1.51812136280714,1.39539254159618,-0.646764802471699));
#23943=CARTESIAN_POINT('Ctrl Pts',(-1.50008999307766,1.35105447038507,-0.687551581002689));
#23944=CARTESIAN_POINT('Ctrl Pts',(-1.48824888379079,1.33182222741682,-0.713138492740816));
#23945=CARTESIAN_POINT('Ctrl Pts',(-1.46055812562105,1.30629366210296,-0.768258557763732));
#23946=CARTESIAN_POINT('Ctrl Pts',(-1.44466308895875,1.3,-0.797770130104052));
#23947=CARTESIAN_POINT('Ctrl Pts',(-1.42894191624432,1.3,-0.825000000000001));
#23948=CARTESIAN_POINT('Ctrl Pts',(-1.28744468918255,1.55,-1.03198167246111));
#23949=CARTESIAN_POINT('Ctrl Pts',(-1.28744468918255,1.58144291640553,-1.03198167246111));
#23950=CARTESIAN_POINT('Ctrl Pts',(-1.29146042158868,1.61494799959182,-1.02703269653942));
#23951=CARTESIAN_POINT('Ctrl Pts',(-1.30734972067592,1.67652816181843,-1.00672880483252));
#23952=CARTESIAN_POINT('Ctrl Pts',(-1.31917543061769,1.70460745840382,-0.991349264982991));
#23953=CARTESIAN_POINT('Ctrl Pts',(-1.34548213209931,1.74894552961493,-0.955340251466734));
#23954=CARTESIAN_POINT('Ctrl Pts',(-1.36172049302549,1.76817777258318,-0.932292094146256));
#23955=CARTESIAN_POINT('Ctrl Pts',(-1.39561049050871,1.79370633789704,-0.880751161609749));
#23956=CARTESIAN_POINT('Ctrl Pts',(-1.4132207435299,1.8,-0.852229869895949));
#23957=CARTESIAN_POINT('Ctrl Pts',(-1.42894191624432,1.8,-0.825000000000001));
#23958=CARTESIAN_POINT('Origin',(0.,1.55,0.));
#23959=CARTESIAN_POINT('',(-1.65,0.85,-2.02066721859313E-16));
#23960=CARTESIAN_POINT('Origin',(0.,0.85,0.));
#23961=CARTESIAN_POINT('',(-1.65,2.25,-2.02066721859313E-16));
#23962=CARTESIAN_POINT('',(-1.65,1.55,-2.02066721859313E-16));
#23963=CARTESIAN_POINT('Origin',(0.,2.25,0.));
#23964=CARTESIAN_POINT('',(-1.42894191624432,1.3,0.825));
#23965=CARTESIAN_POINT('',(-1.42894191624432,1.8,0.825));
#23966=CARTESIAN_POINT('Ctrl Pts',(-1.42894191624432,1.3,0.825));
#23967=CARTESIAN_POINT('Ctrl Pts',(-1.44466308895875,1.3,0.797770130104051));
#23968=CARTESIAN_POINT('Ctrl Pts',(-1.46055812562105,1.30629366210296,0.768258557763731));
#23969=CARTESIAN_POINT('Ctrl Pts',(-1.48824888379079,1.33182222741682,0.713138492740815));
#23970=CARTESIAN_POINT('Ctrl Pts',(-1.50008999307766,1.35105447038507,0.687551581002688));
#23971=CARTESIAN_POINT('Ctrl Pts',(-1.51812136280714,1.39539254159618,0.646764802471698));
#23972=CARTESIAN_POINT('Ctrl Pts',(-1.52552758004446,1.42347183818157,0.628833667319577));
#23973=CARTESIAN_POINT('Ctrl Pts',(-1.53516661651472,1.48505200040818,0.604921184808249));
#23974=CARTESIAN_POINT('Ctrl Pts',(-1.53744468918255,1.51855708359447,0.598968970568895));
#23975=CARTESIAN_POINT('Ctrl Pts',(-1.53744468918255,1.58144291640553,0.598968970568895));
#23976=CARTESIAN_POINT('Ctrl Pts',(-1.53516661651472,1.61494799959182,0.604921184808249));
#23977=CARTESIAN_POINT('Ctrl Pts',(-1.52552758004446,1.67652816181843,0.628833667319577));
#23978=CARTESIAN_POINT('Ctrl Pts',(-1.51812136280714,1.70460745840382,0.646764802471698));
#23979=CARTESIAN_POINT('Ctrl Pts',(-1.50008999307766,1.74894552961493,0.687551581002688));
#23980=CARTESIAN_POINT('Ctrl Pts',(-1.48824888379079,1.76817777258318,0.713138492740815));
#23981=CARTESIAN_POINT('Ctrl Pts',(-1.46055812562105,1.79370633789704,0.768258557763731));
#23982=CARTESIAN_POINT('Ctrl Pts',(-1.44466308895875,1.8,0.797770130104051));
#23983=CARTESIAN_POINT('Ctrl Pts',(-1.42894191624432,1.8,0.825));
#23984=CARTESIAN_POINT('',(-1.28744468918255,1.55,1.03198167246111));
#23985=CARTESIAN_POINT('Ctrl Pts',(-1.42894191624432,1.8,0.825));
#23986=CARTESIAN_POINT('Ctrl Pts',(-1.4132207435299,1.8,0.852229869895948));
#23987=CARTESIAN_POINT('Ctrl Pts',(-1.39561049050871,1.79370633789704,0.880751161609747));
#23988=CARTESIAN_POINT('Ctrl Pts',(-1.36172049302549,1.76817777258318,0.932292094146255));
#23989=CARTESIAN_POINT('Ctrl Pts',(-1.34548213209931,1.74894552961493,0.955340251466733));
#23990=CARTESIAN_POINT('Ctrl Pts',(-1.31917543061769,1.70460745840382,0.991349264982989));
#23991=CARTESIAN_POINT('Ctrl Pts',(-1.30734972067592,1.67652816181843,1.00672880483252));
#23992=CARTESIAN_POINT('Ctrl Pts',(-1.29146042158868,1.61494799959182,1.02703269653942));
#23993=CARTESIAN_POINT('Ctrl Pts',(-1.28744468918255,1.58144291640553,1.03198167246111));
#23994=CARTESIAN_POINT('Ctrl Pts',(-1.28744468918255,1.55,1.03198167246111));
#23995=CARTESIAN_POINT('Ctrl Pts',(-1.28744468918255,1.55,1.03198167246111));
#23996=CARTESIAN_POINT('Ctrl Pts',(-1.28744468918255,1.51855708359447,1.03198167246111));
#23997=CARTESIAN_POINT('Ctrl Pts',(-1.29146042158868,1.48505200040818,1.02703269653942));
#23998=CARTESIAN_POINT('Ctrl Pts',(-1.30734972067592,1.42347183818157,1.00672880483252));
#23999=CARTESIAN_POINT('Ctrl Pts',(-1.31917543061769,1.39539254159618,0.99134926498299));
#24000=CARTESIAN_POINT('Ctrl Pts',(-1.34548213209931,1.35105447038508,0.955340251466733));
#24001=CARTESIAN_POINT('Ctrl Pts',(-1.36172049302549,1.33182222741682,0.932292094146255));
#24002=CARTESIAN_POINT('Ctrl Pts',(-1.39561049050871,1.30629366210296,0.880751161609748));
#24003=CARTESIAN_POINT('Ctrl Pts',(-1.4132207435299,1.3,0.852229869895949));
#24004=CARTESIAN_POINT('Ctrl Pts',(-1.42894191624432,1.3,0.825));
#24005=CARTESIAN_POINT('',(1.42894191624432,1.8,-0.825));
#24006=CARTESIAN_POINT('',(1.42894191624432,1.3,-0.825));
#24007=CARTESIAN_POINT('Ctrl Pts',(1.42894191624432,1.8,-0.825));
#24008=CARTESIAN_POINT('Ctrl Pts',(1.4132207435299,1.8,-0.852229869895949));
#24009=CARTESIAN_POINT('Ctrl Pts',(1.39561049050871,1.79370633789704,-0.880751161609748));
#24010=CARTESIAN_POINT('Ctrl Pts',(1.36172049302549,1.76817777258318,-0.932292094146255));
#24011=CARTESIAN_POINT('Ctrl Pts',(1.34548213209931,1.74894552961493,-0.955340251466734));
#24012=CARTESIAN_POINT('Ctrl Pts',(1.31917543061769,1.70460745840382,-0.99134926498299));
#24013=CARTESIAN_POINT('Ctrl Pts',(1.30734972067592,1.67652816181843,-1.00672880483252));
#24014=CARTESIAN_POINT('Ctrl Pts',(1.29146042158868,1.61494799959182,-1.02703269653942));
#24015=CARTESIAN_POINT('Ctrl Pts',(1.28744468918255,1.58144291640553,-1.03198167246111));
#24016=CARTESIAN_POINT('Ctrl Pts',(1.28744468918255,1.51855708359447,-1.03198167246111));
#24017=CARTESIAN_POINT('Ctrl Pts',(1.29146042158868,1.48505200040818,-1.02703269653942));
#24018=CARTESIAN_POINT('Ctrl Pts',(1.30734972067592,1.42347183818157,-1.00672880483252));
#24019=CARTESIAN_POINT('Ctrl Pts',(1.31917543061769,1.39539254159618,-0.99134926498299));
#24020=CARTESIAN_POINT('Ctrl Pts',(1.34548213209931,1.35105447038507,-0.955340251466734));
#24021=CARTESIAN_POINT('Ctrl Pts',(1.36172049302549,1.33182222741682,-0.932292094146255));
#24022=CARTESIAN_POINT('Ctrl Pts',(1.39561049050871,1.30629366210296,-0.880751161609748));
#24023=CARTESIAN_POINT('Ctrl Pts',(1.4132207435299,1.3,-0.852229869895948));
#24024=CARTESIAN_POINT('Ctrl Pts',(1.42894191624432,1.3,-0.825));
#24025=CARTESIAN_POINT('',(1.53744468918255,1.55,-0.598968970568895));
#24026=CARTESIAN_POINT('Ctrl Pts',(1.42894191624432,1.3,-0.825));
#24027=CARTESIAN_POINT('Ctrl Pts',(1.44466308895875,1.3,-0.797770130104051));
#24028=CARTESIAN_POINT('Ctrl Pts',(1.46055812562105,1.30629366210296,-0.768258557763731));
#24029=CARTESIAN_POINT('Ctrl Pts',(1.48824888379079,1.33182222741682,-0.713138492740815));
#24030=CARTESIAN_POINT('Ctrl Pts',(1.50008999307766,1.35105447038507,-0.687551581002688));
#24031=CARTESIAN_POINT('Ctrl Pts',(1.51812136280714,1.39539254159618,-0.646764802471698));
#24032=CARTESIAN_POINT('Ctrl Pts',(1.52552758004446,1.42347183818157,-0.628833667319577));
#24033=CARTESIAN_POINT('Ctrl Pts',(1.53516661651472,1.48505200040818,-0.604921184808249));
#24034=CARTESIAN_POINT('Ctrl Pts',(1.53744468918255,1.51855708359447,-0.598968970568895));
#24035=CARTESIAN_POINT('Ctrl Pts',(1.53744468918255,1.55,-0.598968970568895));
#24036=CARTESIAN_POINT('Ctrl Pts',(1.53744468918255,1.55,-0.598968970568895));
#24037=CARTESIAN_POINT('Ctrl Pts',(1.53744468918255,1.58144291640553,-0.598968970568895));
#24038=CARTESIAN_POINT('Ctrl Pts',(1.53516661651472,1.61494799959182,-0.604921184808249));
#24039=CARTESIAN_POINT('Ctrl Pts',(1.52552758004446,1.67652816181843,-0.628833667319577));
#24040=CARTESIAN_POINT('Ctrl Pts',(1.51812136280714,1.70460745840382,-0.646764802471698));
#24041=CARTESIAN_POINT('Ctrl Pts',(1.50008999307766,1.74894552961493,-0.687551581002688));
#24042=CARTESIAN_POINT('Ctrl Pts',(1.48824888379079,1.76817777258318,-0.713138492740815));
#24043=CARTESIAN_POINT('Ctrl Pts',(1.46055812562105,1.79370633789704,-0.768258557763731));
#24044=CARTESIAN_POINT('Ctrl Pts',(1.44466308895875,1.8,-0.797770130104051));
#24045=CARTESIAN_POINT('Ctrl Pts',(1.42894191624432,1.8,-0.825));
#24046=CARTESIAN_POINT('',(0.,1.3,-1.65));
#24047=CARTESIAN_POINT('',(0.,1.8,-1.65));
#24048=CARTESIAN_POINT('Ctrl Pts',(1.38777878078145E-17,1.3,-1.65));
#24049=CARTESIAN_POINT('Ctrl Pts',(0.0314423454288489,1.3,-1.65));
#24050=CARTESIAN_POINT('Ctrl Pts',(0.0649476351123396,1.30629366210296,
-1.64900971937348));
#24051=CARTESIAN_POINT('Ctrl Pts',(0.126528390765307,1.33182222741682,-1.64543058688707));
#24052=CARTESIAN_POINT('Ctrl Pts',(0.154607860978348,1.35105447038507,-1.64289183246942));
#24053=CARTESIAN_POINT('Ctrl Pts',(0.198945932189457,1.39539254159618,-1.63811406745469));
#24054=CARTESIAN_POINT('Ctrl Pts',(0.218177859368546,1.42347183818157,-1.63556247215209));
#24055=CARTESIAN_POINT('Ctrl Pts',(0.243706194926033,1.48505200040818,-1.63195388134767));
#24056=CARTESIAN_POINT('Ctrl Pts',(0.25,1.51855708359447,-1.63095064303001));
#24057=CARTESIAN_POINT('Ctrl Pts',(0.25,1.58144291640553,-1.63095064303001));
#24058=CARTESIAN_POINT('Ctrl Pts',(0.243706194926033,1.61494799959182,-1.63195388134767));
#24059=CARTESIAN_POINT('Ctrl Pts',(0.218177859368546,1.67652816181843,-1.63556247215209));
#24060=CARTESIAN_POINT('Ctrl Pts',(0.198945932189457,1.70460745840382,-1.63811406745469));
#24061=CARTESIAN_POINT('Ctrl Pts',(0.154607860978349,1.74894552961493,-1.64289183246942));
#24062=CARTESIAN_POINT('Ctrl Pts',(0.126528390765307,1.76817777258318,-1.64543058688707));
#24063=CARTESIAN_POINT('Ctrl Pts',(0.0649476351123398,1.79370633789704,
-1.64900971937348));
#24064=CARTESIAN_POINT('Ctrl Pts',(0.031442345428849,1.8,-1.65));
#24065=CARTESIAN_POINT('Ctrl Pts',(7.63278329429795E-17,1.8,-1.65));
#24066=CARTESIAN_POINT('',(-0.25,1.55,-1.63095064303001));
#24067=CARTESIAN_POINT('Ctrl Pts',(9.0205620750794E-17,1.8,-1.65));
#24068=CARTESIAN_POINT('Ctrl Pts',(-0.0314423454288488,1.8,-1.65));
#24069=CARTESIAN_POINT('Ctrl Pts',(-0.0649476351123396,1.79370633789704,
-1.64900971937348));
#24070=CARTESIAN_POINT('Ctrl Pts',(-0.126528390765307,1.76817777258318,
-1.64543058688707));
#24071=CARTESIAN_POINT('Ctrl Pts',(-0.154607860978348,1.74894552961493,
-1.64289183246942));
#24072=CARTESIAN_POINT('Ctrl Pts',(-0.198945932189456,1.70460745840382,
-1.63811406745469));
#24073=CARTESIAN_POINT('Ctrl Pts',(-0.218177859368546,1.67652816181843,
-1.63556247215209));
#24074=CARTESIAN_POINT('Ctrl Pts',(-0.243706194926033,1.61494799959182,
-1.63195388134767));
#24075=CARTESIAN_POINT('Ctrl Pts',(-0.25,1.58144291640553,-1.63095064303001));
#24076=CARTESIAN_POINT('Ctrl Pts',(-0.25,1.55,-1.63095064303001));
#24077=CARTESIAN_POINT('Ctrl Pts',(-0.25,1.55,-1.63095064303001));
#24078=CARTESIAN_POINT('Ctrl Pts',(-0.25,1.51855708359447,-1.63095064303001));
#24079=CARTESIAN_POINT('Ctrl Pts',(-0.243706194926033,1.48505200040818,
-1.63195388134767));
#24080=CARTESIAN_POINT('Ctrl Pts',(-0.218177859368546,1.42347183818157,
-1.63556247215209));
#24081=CARTESIAN_POINT('Ctrl Pts',(-0.198945932189457,1.39539254159618,
-1.63811406745469));
#24082=CARTESIAN_POINT('Ctrl Pts',(-0.154607860978349,1.35105447038507,
-1.64289183246942));
#24083=CARTESIAN_POINT('Ctrl Pts',(-0.126528390765307,1.33182222741682,
-1.64543058688707));
#24084=CARTESIAN_POINT('Ctrl Pts',(-0.0649476351123398,1.30629366210296,
-1.64900971937348));
#24085=CARTESIAN_POINT('Ctrl Pts',(-0.031442345428849,1.3,-1.65));
#24086=CARTESIAN_POINT('Ctrl Pts',(-4.85722573273506E-17,1.3,-1.65));
#24087=CARTESIAN_POINT('',(0.,1.8,1.65));
#24088=CARTESIAN_POINT('',(0.,1.3,1.65));
#24089=CARTESIAN_POINT('Ctrl Pts',(8.32667268468867E-17,1.8,1.65));
#24090=CARTESIAN_POINT('Ctrl Pts',(0.031442345428849,1.8,1.65));
#24091=CARTESIAN_POINT('Ctrl Pts',(0.0649476351123398,1.79370633789704,
1.64900971937348));
#24092=CARTESIAN_POINT('Ctrl Pts',(0.126528390765307,1.76817777258318,1.64543058688707));
#24093=CARTESIAN_POINT('Ctrl Pts',(0.154607860978349,1.74894552961493,1.64289183246942));
#24094=CARTESIAN_POINT('Ctrl Pts',(0.198945932189457,1.70460745840382,1.63811406745469));
#24095=CARTESIAN_POINT('Ctrl Pts',(0.218177859368546,1.67652816181843,1.63556247215209));
#24096=CARTESIAN_POINT('Ctrl Pts',(0.243706194926033,1.61494799959182,1.63195388134767));
#24097=CARTESIAN_POINT('Ctrl Pts',(0.25,1.58144291640553,1.63095064303001));
#24098=CARTESIAN_POINT('Ctrl Pts',(0.25,1.51855708359447,1.63095064303001));
#24099=CARTESIAN_POINT('Ctrl Pts',(0.243706194926033,1.48505200040818,1.63195388134767));
#24100=CARTESIAN_POINT('Ctrl Pts',(0.218177859368546,1.42347183818157,1.63556247215209));
#24101=CARTESIAN_POINT('Ctrl Pts',(0.198945932189457,1.39539254159618,1.63811406745469));
#24102=CARTESIAN_POINT('Ctrl Pts',(0.154607860978348,1.35105447038507,1.64289183246942));
#24103=CARTESIAN_POINT('Ctrl Pts',(0.126528390765307,1.33182222741682,1.64543058688707));
#24104=CARTESIAN_POINT('Ctrl Pts',(0.0649476351123397,1.30629366210296,
1.64900971937348));
#24105=CARTESIAN_POINT('Ctrl Pts',(0.0314423454288488,1.3,1.65));
#24106=CARTESIAN_POINT('Ctrl Pts',(-1.38777878078145E-17,1.3,1.65));
#24107=CARTESIAN_POINT('',(-0.25,1.55,1.63095064303001));
#24108=CARTESIAN_POINT('Ctrl Pts',(-5.55111512312578E-17,1.3,1.65));
#24109=CARTESIAN_POINT('Ctrl Pts',(-0.031442345428849,1.3,1.65));
#24110=CARTESIAN_POINT('Ctrl Pts',(-0.0649476351123398,1.30629366210296,
1.64900971937348));
#24111=CARTESIAN_POINT('Ctrl Pts',(-0.126528390765307,1.33182222741682,
1.64543058688707));
#24112=CARTESIAN_POINT('Ctrl Pts',(-0.154607860978349,1.35105447038507,
1.64289183246942));
#24113=CARTESIAN_POINT('Ctrl Pts',(-0.198945932189457,1.39539254159618,
1.63811406745469));
#24114=CARTESIAN_POINT('Ctrl Pts',(-0.218177859368546,1.42347183818157,
1.63556247215209));
#24115=CARTESIAN_POINT('Ctrl Pts',(-0.243706194926033,1.48505200040818,
1.63195388134767));
#24116=CARTESIAN_POINT('Ctrl Pts',(-0.25,1.51855708359447,1.63095064303001));
#24117=CARTESIAN_POINT('Ctrl Pts',(-0.25,1.55,1.63095064303001));
#24118=CARTESIAN_POINT('Ctrl Pts',(-0.25,1.55,1.63095064303001));
#24119=CARTESIAN_POINT('Ctrl Pts',(-0.25,1.58144291640553,1.63095064303001));
#24120=CARTESIAN_POINT('Ctrl Pts',(-0.243706194926033,1.61494799959182,
1.63195388134767));
#24121=CARTESIAN_POINT('Ctrl Pts',(-0.218177859368546,1.67652816181843,
1.63556247215209));
#24122=CARTESIAN_POINT('Ctrl Pts',(-0.198945932189456,1.70460745840382,
1.63811406745469));
#24123=CARTESIAN_POINT('Ctrl Pts',(-0.154607860978348,1.74894552961493,
1.64289183246942));
#24124=CARTESIAN_POINT('Ctrl Pts',(-0.126528390765307,1.76817777258318,
1.64543058688707));
#24125=CARTESIAN_POINT('Ctrl Pts',(-0.0649476351123396,1.79370633789704,
1.64900971937348));
#24126=CARTESIAN_POINT('Ctrl Pts',(-0.0314423454288488,1.8,1.65));
#24127=CARTESIAN_POINT('Ctrl Pts',(7.63278329429795E-17,1.8,1.65));
#24128=CARTESIAN_POINT('Origin',(0.,1.55,0.));
#24129=CARTESIAN_POINT('',(-0.713525491562421,1.55,0.700629269222037));
#24130=CARTESIAN_POINT('',(0.125,1.55,0.21650635094611));
#24131=CARTESIAN_POINT('Ctrl Pts',(-0.713525491562421,1.55,0.700629269222037));
#24132=CARTESIAN_POINT('Ctrl Pts',(-0.713525491562421,1.5815373526696,0.700629269222037));
#24133=CARTESIAN_POINT('Ctrl Pts',(-0.718163997970498,1.61508042700263,
0.695997784676727));
#24134=CARTESIAN_POINT('Ctrl Pts',(-0.73619249062986,1.67663267125761,0.676899590973058));
#24135=CARTESIAN_POINT('Ctrl Pts',(-0.749495710301795,1.70465411363682,
0.662390652284073));
#24136=CARTESIAN_POINT('Ctrl Pts',(-0.778498278845144,1.74889618382539,
0.628048950774009));
#24137=CARTESIAN_POINT('Ctrl Pts',(-0.796153444118959,1.76811531482682,
0.605884303066698));
#24138=CARTESIAN_POINT('Ctrl Pts',(-0.832065554235658,1.79367084275751,
0.555538485325663));
#24139=CARTESIAN_POINT('Ctrl Pts',(-0.850258932191534,1.8,0.527308329855002));
#24140=CARTESIAN_POINT('Ctrl Pts',(-0.881791875377343,1.8,0.472691670144998));
#24141=CARTESIAN_POINT('Ctrl Pts',(-0.897143218189782,1.79367084275751,
0.442820664919227));
#24142=CARTESIAN_POINT('Ctrl Pts',(-0.92278792026947,1.76811531482682,0.386546956384144));
#24143=CARTESIAN_POINT('Ctrl Pts',(-0.933155485613026,1.74889618382539,
0.360174810895352));
#24144=CARTESIAN_POINT('Ctrl Pts',(-0.948394987258249,1.70465411363682,
0.31788699900678));
#24145=CARTESIAN_POINT('Ctrl Pts',(-0.954308486908894,1.67663267125761,
0.299111603474267));
#24146=CARTESIAN_POINT('Ctrl Pts',(-0.961833761492987,1.61508042700263,
0.273949373987484));
#24147=CARTESIAN_POINT('Ctrl Pts',(-0.963525491562421,1.5815373526696,0.267616567329817));
#24148=CARTESIAN_POINT('Ctrl Pts',(-0.963525491562421,1.5184626473304,0.267616567329817));
#24149=CARTESIAN_POINT('Ctrl Pts',(-0.961833761492987,1.48491957299737,
0.273949373987484));
#24150=CARTESIAN_POINT('Ctrl Pts',(-0.954308486908894,1.42336732874239,
0.299111603474267));
#24151=CARTESIAN_POINT('Ctrl Pts',(-0.948394987258249,1.39534588636318,
0.31788699900678));
#24152=CARTESIAN_POINT('Ctrl Pts',(-0.933155485613026,1.35110381617461,
0.360174810895352));
#24153=CARTESIAN_POINT('Ctrl Pts',(-0.92278792026947,1.33188468517318,0.386546956384144));
#24154=CARTESIAN_POINT('Ctrl Pts',(-0.897143218189782,1.30632915724249,
0.442820664919227));
#24155=CARTESIAN_POINT('Ctrl Pts',(-0.881791875377343,1.3,0.472691670144998));
#24156=CARTESIAN_POINT('Ctrl Pts',(-0.850258932191534,1.3,0.527308329855002));
#24157=CARTESIAN_POINT('Ctrl Pts',(-0.832065554235658,1.30632915724249,
0.555538485325663));
#24158=CARTESIAN_POINT('Ctrl Pts',(-0.796153444118959,1.33188468517318,
0.605884303066698));
#24159=CARTESIAN_POINT('Ctrl Pts',(-0.778498278845144,1.35110381617461,
0.628048950774009));
#24160=CARTESIAN_POINT('Ctrl Pts',(-0.749495710301795,1.39534588636318,
0.662390652284073));
#24161=CARTESIAN_POINT('Ctrl Pts',(-0.73619249062986,1.42336732874239,0.676899590973058));
#24162=CARTESIAN_POINT('Ctrl Pts',(-0.718163997970498,1.48491957299737,
0.695997784676727));
#24163=CARTESIAN_POINT('Ctrl Pts',(-0.713525491562421,1.5184626473304,0.700629269222037));
#24164=CARTESIAN_POINT('Ctrl Pts',(-0.713525491562421,1.55,0.700629269222037));
#24165=CARTESIAN_POINT('Origin',(0.,1.55,0.));
#24166=CARTESIAN_POINT('',(0.963525491562421,1.55,-0.267616567329817));
#24167=CARTESIAN_POINT('Ctrl Pts',(0.963525491562421,1.55,-0.267616567329817));
#24168=CARTESIAN_POINT('Ctrl Pts',(0.963525491562421,1.5184626473304,-0.267616567329817));
#24169=CARTESIAN_POINT('Ctrl Pts',(0.961833761492987,1.48491957299737,-0.273949373987484));
#24170=CARTESIAN_POINT('Ctrl Pts',(0.954308486908894,1.42336732874239,-0.299111603474267));
#24171=CARTESIAN_POINT('Ctrl Pts',(0.948394987258249,1.39534588636318,-0.31788699900678));
#24172=CARTESIAN_POINT('Ctrl Pts',(0.933155485613026,1.35110381617461,-0.360174810895352));
#24173=CARTESIAN_POINT('Ctrl Pts',(0.92278792026947,1.33188468517318,-0.386546956384144));
#24174=CARTESIAN_POINT('Ctrl Pts',(0.897143218189782,1.30632915724249,-0.442820664919227));
#24175=CARTESIAN_POINT('Ctrl Pts',(0.881791875377343,1.3,-0.472691670144998));
#24176=CARTESIAN_POINT('Ctrl Pts',(0.850258932191534,1.3,-0.527308329855002));
#24177=CARTESIAN_POINT('Ctrl Pts',(0.832065554235658,1.30632915724249,-0.555538485325663));
#24178=CARTESIAN_POINT('Ctrl Pts',(0.796153444118959,1.33188468517318,-0.605884303066698));
#24179=CARTESIAN_POINT('Ctrl Pts',(0.778498278845144,1.35110381617461,-0.628048950774009));
#24180=CARTESIAN_POINT('Ctrl Pts',(0.749495710301795,1.39534588636318,-0.662390652284073));
#24181=CARTESIAN_POINT('Ctrl Pts',(0.73619249062986,1.42336732874239,-0.676899590973058));
#24182=CARTESIAN_POINT('Ctrl Pts',(0.718163997970498,1.48491957299737,-0.695997784676727));
#24183=CARTESIAN_POINT('Ctrl Pts',(0.713525491562421,1.5184626473304,-0.700629269222037));
#24184=CARTESIAN_POINT('Ctrl Pts',(0.713525491562421,1.5815373526696,-0.700629269222037));
#24185=CARTESIAN_POINT('Ctrl Pts',(0.718163997970498,1.61508042700263,-0.695997784676727));
#24186=CARTESIAN_POINT('Ctrl Pts',(0.73619249062986,1.67663267125761,-0.676899590973058));
#24187=CARTESIAN_POINT('Ctrl Pts',(0.749495710301795,1.70465411363682,-0.662390652284073));
#24188=CARTESIAN_POINT('Ctrl Pts',(0.778498278845144,1.74889618382539,-0.628048950774009));
#24189=CARTESIAN_POINT('Ctrl Pts',(0.796153444118959,1.76811531482682,-0.605884303066698));
#24190=CARTESIAN_POINT('Ctrl Pts',(0.832065554235658,1.79367084275751,-0.555538485325663));
#24191=CARTESIAN_POINT('Ctrl Pts',(0.850258932191534,1.8,-0.527308329855002));
#24192=CARTESIAN_POINT('Ctrl Pts',(0.881791875377343,1.8,-0.472691670144998));
#24193=CARTESIAN_POINT('Ctrl Pts',(0.897143218189782,1.79367084275751,-0.442820664919227));
#24194=CARTESIAN_POINT('Ctrl Pts',(0.92278792026947,1.76811531482682,-0.386546956384144));
#24195=CARTESIAN_POINT('Ctrl Pts',(0.933155485613026,1.74889618382539,-0.360174810895352));
#24196=CARTESIAN_POINT('Ctrl Pts',(0.948394987258249,1.70465411363682,-0.31788699900678));
#24197=CARTESIAN_POINT('Ctrl Pts',(0.954308486908894,1.67663267125761,-0.299111603474267));
#24198=CARTESIAN_POINT('Ctrl Pts',(0.961833761492987,1.61508042700263,-0.273949373987484));
#24199=CARTESIAN_POINT('Ctrl Pts',(0.963525491562421,1.5815373526696,-0.267616567329817));
#24200=CARTESIAN_POINT('Ctrl Pts',(0.963525491562421,1.55,-0.267616567329817));
#24201=CARTESIAN_POINT('',(0.125,1.55,0.21650635094611));
#24202=CARTESIAN_POINT('Origin',(0.,1.55,0.));
#24203=CARTESIAN_POINT('',(-0.25,1.55,-0.968245836551854));
#24204=CARTESIAN_POINT('',(-0.25,1.55,0.));
#24205=CARTESIAN_POINT('Ctrl Pts',(-0.25,1.55,-0.968245836551854));
#24206=CARTESIAN_POINT('Ctrl Pts',(-0.25,1.5815373526696,-0.968245836551854));
#24207=CARTESIAN_POINT('Ctrl Pts',(-0.243669763522489,1.61508042700263,
-0.969947158664211));
#24208=CARTESIAN_POINT('Ctrl Pts',(-0.218115996279034,1.67663267125761,
-0.976011194447325));
#24209=CARTESIAN_POINT('Ctrl Pts',(-0.198899276956455,1.70465411363682,
-0.980277651290853));
#24210=CARTESIAN_POINT('Ctrl Pts',(-0.154657206767882,1.74889618382539,
-0.988223761669361));
#24211=CARTESIAN_POINT('Ctrl Pts',(-0.126634476150511,1.76811531482682,
-0.992431259450842));
#24212=CARTESIAN_POINT('Ctrl Pts',(-0.0650776639541238,1.79367084275751,
-0.99835915024489));
#24213=CARTESIAN_POINT('Ctrl Pts',(-0.0315329431858092,1.8,-1.));
#24214=CARTESIAN_POINT('Ctrl Pts',(0.0315329431858092,1.8,-1.));
#24215=CARTESIAN_POINT('Ctrl Pts',(0.0650776639541238,1.79367084275751,
-0.99835915024489));
#24216=CARTESIAN_POINT('Ctrl Pts',(0.126634476150511,1.76811531482682,-0.992431259450842));
#24217=CARTESIAN_POINT('Ctrl Pts',(0.154657206767882,1.74889618382539,-0.988223761669361));
#24218=CARTESIAN_POINT('Ctrl Pts',(0.198899276956455,1.70465411363682,-0.980277651290853));
#24219=CARTESIAN_POINT('Ctrl Pts',(0.218115996279034,1.67663267125761,-0.976011194447325));
#24220=CARTESIAN_POINT('Ctrl Pts',(0.243669763522488,1.61508042700263,-0.969947158664211));
#24221=CARTESIAN_POINT('Ctrl Pts',(0.25,1.5815373526696,-0.968245836551854));
#24222=CARTESIAN_POINT('Ctrl Pts',(0.25,1.5184626473304,-0.968245836551854));
#24223=CARTESIAN_POINT('Ctrl Pts',(0.243669763522488,1.48491957299737,-0.969947158664211));
#24224=CARTESIAN_POINT('Ctrl Pts',(0.218115996279034,1.42336732874239,-0.976011194447325));
#24225=CARTESIAN_POINT('Ctrl Pts',(0.198899276956455,1.39534588636318,-0.980277651290853));
#24226=CARTESIAN_POINT('Ctrl Pts',(0.154657206767882,1.35110381617461,-0.988223761669361));
#24227=CARTESIAN_POINT('Ctrl Pts',(0.126634476150511,1.33188468517318,-0.992431259450842));
#24228=CARTESIAN_POINT('Ctrl Pts',(0.0650776639541239,1.30632915724249,
-0.99835915024489));
#24229=CARTESIAN_POINT('Ctrl Pts',(0.0315329431858092,1.3,-1.));
#24230=CARTESIAN_POINT('Ctrl Pts',(-0.0315329431858092,1.3,-1.));
#24231=CARTESIAN_POINT('Ctrl Pts',(-0.0650776639541239,1.30632915724249,
-0.99835915024489));
#24232=CARTESIAN_POINT('Ctrl Pts',(-0.126634476150511,1.33188468517318,
-0.992431259450842));
#24233=CARTESIAN_POINT('Ctrl Pts',(-0.154657206767882,1.35110381617461,
-0.988223761669361));
#24234=CARTESIAN_POINT('Ctrl Pts',(-0.198899276956455,1.39534588636318,
-0.980277651290853));
#24235=CARTESIAN_POINT('Ctrl Pts',(-0.218115996279034,1.42336732874239,
-0.976011194447325));
#24236=CARTESIAN_POINT('Ctrl Pts',(-0.243669763522489,1.48491957299737,
-0.969947158664211));
#24237=CARTESIAN_POINT('Ctrl Pts',(-0.25,1.5184626473304,-0.968245836551854));
#24238=CARTESIAN_POINT('Ctrl Pts',(-0.25,1.55,-0.968245836551854));
#24239=CARTESIAN_POINT('Origin',(0.,1.55,0.));
#24240=CARTESIAN_POINT('',(-0.25,1.55,0.968245836551854));
#24241=CARTESIAN_POINT('Ctrl Pts',(-0.25,1.55,0.968245836551854));
#24242=CARTESIAN_POINT('Ctrl Pts',(-0.25,1.5184626473304,0.968245836551854));
#24243=CARTESIAN_POINT('Ctrl Pts',(-0.243669763522489,1.48491957299737,
0.969947158664211));
#24244=CARTESIAN_POINT('Ctrl Pts',(-0.218115996279034,1.42336732874239,
0.976011194447325));
#24245=CARTESIAN_POINT('Ctrl Pts',(-0.198899276956455,1.39534588636318,
0.980277651290853));
#24246=CARTESIAN_POINT('Ctrl Pts',(-0.154657206767882,1.35110381617461,
0.988223761669361));
#24247=CARTESIAN_POINT('Ctrl Pts',(-0.126634476150511,1.33188468517318,
0.992431259450842));
#24248=CARTESIAN_POINT('Ctrl Pts',(-0.065077663954124,1.30632915724249,
0.99835915024489));
#24249=CARTESIAN_POINT('Ctrl Pts',(-0.0315329431858092,1.3,1.));
#24250=CARTESIAN_POINT('Ctrl Pts',(0.0315329431858092,1.3,1.));
#24251=CARTESIAN_POINT('Ctrl Pts',(0.065077663954124,1.30632915724249,0.99835915024489));
#24252=CARTESIAN_POINT('Ctrl Pts',(0.126634476150511,1.33188468517318,0.992431259450842));
#24253=CARTESIAN_POINT('Ctrl Pts',(0.154657206767882,1.35110381617461,0.988223761669361));
#24254=CARTESIAN_POINT('Ctrl Pts',(0.198899276956455,1.39534588636318,0.980277651290853));
#24255=CARTESIAN_POINT('Ctrl Pts',(0.218115996279034,1.42336732874239,0.976011194447325));
#24256=CARTESIAN_POINT('Ctrl Pts',(0.243669763522488,1.48491957299737,0.969947158664211));
#24257=CARTESIAN_POINT('Ctrl Pts',(0.25,1.5184626473304,0.968245836551854));
#24258=CARTESIAN_POINT('Ctrl Pts',(0.25,1.5815373526696,0.968245836551854));
#24259=CARTESIAN_POINT('Ctrl Pts',(0.243669763522488,1.61508042700263,0.969947158664211));
#24260=CARTESIAN_POINT('Ctrl Pts',(0.218115996279034,1.67663267125761,0.976011194447325));
#24261=CARTESIAN_POINT('Ctrl Pts',(0.198899276956455,1.70465411363682,0.980277651290853));
#24262=CARTESIAN_POINT('Ctrl Pts',(0.154657206767882,1.74889618382539,0.988223761669361));
#24263=CARTESIAN_POINT('Ctrl Pts',(0.126634476150511,1.76811531482682,0.992431259450842));
#24264=CARTESIAN_POINT('Ctrl Pts',(0.0650776639541239,1.79367084275751,
0.99835915024489));
#24265=CARTESIAN_POINT('Ctrl Pts',(0.0315329431858092,1.8,1.));
#24266=CARTESIAN_POINT('Ctrl Pts',(-0.0315329431858092,1.8,1.));
#24267=CARTESIAN_POINT('Ctrl Pts',(-0.0650776639541239,1.79367084275751,
0.99835915024489));
#24268=CARTESIAN_POINT('Ctrl Pts',(-0.126634476150511,1.76811531482682,
0.992431259450842));
#24269=CARTESIAN_POINT('Ctrl Pts',(-0.154657206767882,1.74889618382539,
0.988223761669361));
#24270=CARTESIAN_POINT('Ctrl Pts',(-0.198899276956455,1.70465411363682,
0.980277651290853));
#24271=CARTESIAN_POINT('Ctrl Pts',(-0.218115996279034,1.67663267125761,
0.976011194447325));
#24272=CARTESIAN_POINT('Ctrl Pts',(-0.243669763522489,1.61508042700263,
0.969947158664211));
#24273=CARTESIAN_POINT('Ctrl Pts',(-0.25,1.5815373526696,0.968245836551854));
#24274=CARTESIAN_POINT('Ctrl Pts',(-0.25,1.55,0.968245836551854));
#24275=CARTESIAN_POINT('',(-0.25,1.55,0.));
#24276=CARTESIAN_POINT('Origin',(1.65,2.25,0.));
#24277=CARTESIAN_POINT('',(-1.,2.25,-1.22464679914735E-16));
#24278=CARTESIAN_POINT('Origin',(0.,2.25,0.));
#24279=CARTESIAN_POINT('Origin',(1.75,0.85,0.));
#24280=CARTESIAN_POINT('',(-1.75,0.85,-2.14313189850787E-16));
#24281=CARTESIAN_POINT('Origin',(0.,0.85,0.));
#24282=CARTESIAN_POINT('Origin',(0.,0.,0.));
#24283=CARTESIAN_POINT('',(-1.75,-0.85,-2.14313189850787E-16));
#24284=CARTESIAN_POINT('Origin',(0.,-0.85,0.));
#24285=CARTESIAN_POINT('',(-1.75,0.,-2.14313189850787E-16));
#24286=CARTESIAN_POINT('Origin',(1.,-0.85,0.));
#24287=CARTESIAN_POINT('',(-1.,-0.85,-1.22464679914735E-16));
#24288=CARTESIAN_POINT('Origin',(0.,-0.85,0.));
#24289=CARTESIAN_POINT('Origin',(0.,0.7,0.));
#24290=CARTESIAN_POINT('',(-1.,0.7,-1.22464679914735E-16));
#26961=UNCERTAINTY_MEASURE_WITH_UNIT(LENGTH_MEASURE(0.001),#27070,
'DISTANCE_ACCURACY_VALUE',
'Maximum model space distance between geometric entities at asserted c
onnectivities');
#26992=UNCERTAINTY_MEASURE_WITH_UNIT(LENGTH_MEASURE(0.001),#27070,
'DISTANCE_ACCURACY_VALUE',
'Maximum model space distance between geometric entities at asserted c
onnectivities');
#27038=(
GEOMETRIC_REPRESENTATION_CONTEXT(3)
GLOBAL_UNCERTAINTY_ASSIGNED_CONTEXT((#26961))
GLOBAL_UNIT_ASSIGNED_CONTEXT((#27070,#27072,#27073))
REPRESENTATION_CONTEXT('','3D')
);
#27069=(
GEOMETRIC_REPRESENTATION_CONTEXT(3)
GLOBAL_UNCERTAINTY_ASSIGNED_CONTEXT((#26992))
GLOBAL_UNIT_ASSIGNED_CONTEXT((#27070,#27072,#27073))
REPRESENTATION_CONTEXT('','3D')
);
#27070=(
LENGTH_UNIT()
NAMED_UNIT(*)
SI_UNIT(.CENTI.,.METRE.)
);
#27072=(
NAMED_UNIT(*)
PLANE_ANGLE_UNIT()
SI_UNIT($,.RADIAN.)
);
#27073=(
NAMED_UNIT(*)
SI_UNIT($,.STERADIAN.)
SOLID_ANGLE_UNIT()
);
#27119=SHAPE_DEFINITION_REPRESENTATION(#27205,#27396);
#27205=PRODUCT_DEFINITION_SHAPE('',$,#27473);
#27396=SHAPE_REPRESENTATION('',(#15549),#27038);
#27427=PRODUCT_DEFINITION_CONTEXT('part definition',#27657,'design');
#27473=PRODUCT_DEFINITION('Insert bearing','Insert bearing',#27549,#27427);
#27549=PRODUCT_DEFINITION_FORMATION('',$,#27704);
#27657=APPLICATION_CONTEXT(
'Core Data for Automotive Mechanical Design Process');
#27658=PRODUCT_CONTEXT('part definition',#27657,'mechanical');
#27704=PRODUCT('Insert bearing','Insert bearing','Insert bearing',(#27658));
#27791=COLOUR_RGB('Grey',0.48,0.52,0.57);
#27792=FILL_AREA_STYLE_COLOUR('',#27791);
#27793=FILL_AREA_STYLE('',(#27792));
#27794=SURFACE_STYLE_FILL_AREA(#27793);
#27795=SURFACE_SIDE_STYLE('',(#27794));
#27796=SURFACE_STYLE_USAGE(.BOTH.,#27795);
#27797=PRESENTATION_STYLE_ASSIGNMENT((#27796));
ENDSEC;
END-ISO-10303-21;
